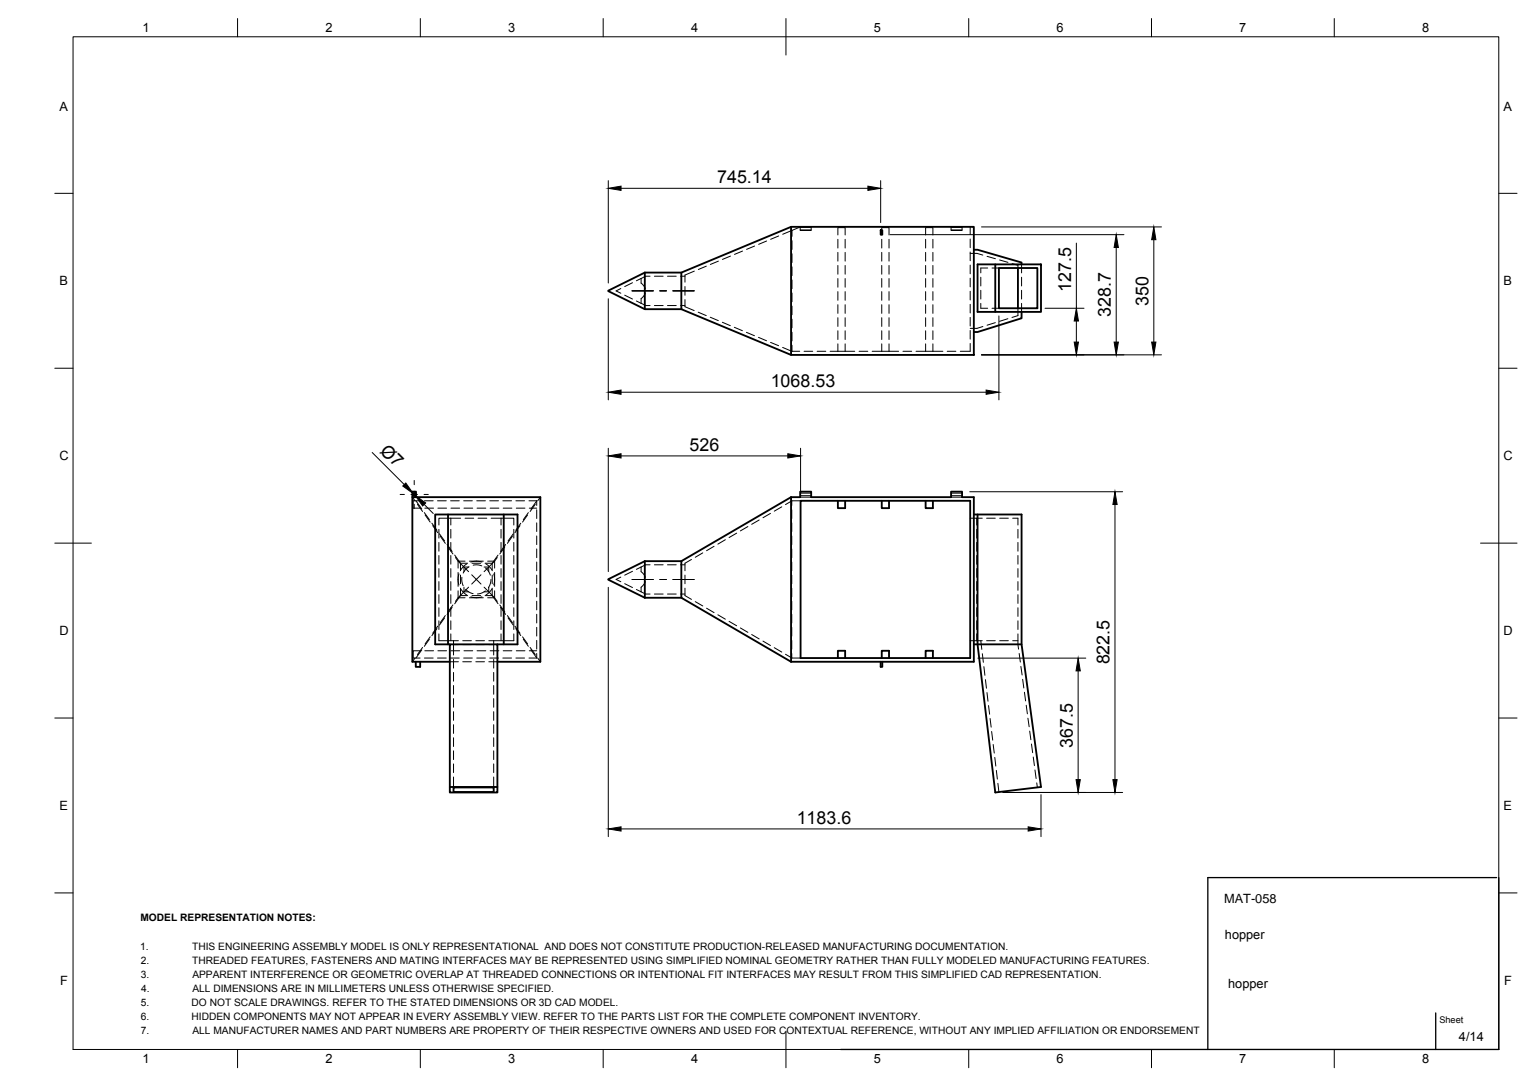
ISO-10303-21;
HEADER;
FILE_DESCRIPTION (('STEP AP214'),
    '1' );
FILE_NAME ('hopper.step',
    '2026-10-21T17:54:40',
    ( '' ),
    ( '' ),
    'SwSTEP 2.0',
    'SolidWorks 2026',
    '' );
FILE_SCHEMA (( 'AUTOMOTIVE_DESIGN' ));
ENDSEC;

DATA;
#6=ADVANCED_FACE ( 'NONE', ( #30321 ), #29814, .T. ) ;
#33=VECTOR ( 'NONE', #35078, 1000.000000000000000 ) ;
#69=AXIS2_PLACEMENT_3D ( 'NONE', #31209, #39422, #27614 ) ;
#97=LINE ( 'NONE', #40110, #967 ) ;
#99=ORIENTED_EDGE ( 'NONE', *, *, #35916, .T. ) ;
#106=CARTESIAN_POINT ( 'NONE',  ( -194.9999999999999432, 173.0000000000000000, 372.0000000000000000 ) ) ;
#168=ADVANCED_FACE ( 'NONE', ( #34691 ), #50265, .F. ) ;
#187=CARTESIAN_POINT ( 'NONE',  ( 214.9999999999999432, 164.9999999999999716, 132.0000000000000000 ) ) ;
#200=DIRECTION ( 'NONE',  ( -0.000000000000000000, -0.000000000000000000, 1.000000000000000000 ) ) ;
#209=VECTOR ( 'NONE', #36714, 1000.000000000000000 ) ;
#234=DIRECTION ( 'NONE',  ( -0.8962124318248270161, 0.000000000000000000, 0.4436251537532894806 ) ) ;
#244=PLANE ( 'NONE',  #29355 ) ;
#300=EDGE_CURVE ( 'NONE', #33060, #42445, #25916, .T. ) ;
#327=DIRECTION ( 'NONE',  ( 1.000000000000000000, 0.000000000000000000, -0.000000000000000000 ) ) ;
#337=CARTESIAN_POINT ( 'NONE',  ( 0.000000000000000000, 0.000000000000000000, 910.0000000000000000 ) ) ;
#341=PLANE ( 'NONE',  #14465 ) ;
#350=DIRECTION ( 'NONE',  ( -1.000000000000000000, -0.000000000000000000, -0.000000000000000000 ) ) ;
#356=DIRECTION ( 'NONE',  ( 0.000000000000000000, -1.000000000000000000, 0.000000000000000000 ) ) ;
#365=ORIENTED_EDGE ( 'NONE', *, *, #8301, .F. ) ;
#366=DIRECTION ( 'NONE',  ( 1.000000000000000000, 0.000000000000000000, 0.000000000000000000 ) ) ;
#369=CARTESIAN_POINT ( 'NONE',  ( -225.0000000000000568, -165.6999999999999602, 254.8599999999999852 ) ) ;
#377=DIRECTION ( 'NONE',  ( 0.000000000000000000, -0.000000000000000000, -1.000000000000000000 ) ) ;
#378=CARTESIAN_POINT ( 'NONE',  ( 0.5000000000000000000, -0.5000000000000000000, 1000.000000000000000 ) ) ;
#386=CARTESIAN_POINT ( 'NONE',  ( 0.000000000000000000, 0.000000000000000000, 910.0000000000000000 ) ) ;
#398=ORIENTED_EDGE ( 'NONE', *, *, #44450, .F. ) ;
#403=EDGE_LOOP ( 'NONE', ( #46548, #45741, #3676, #28607 ) ) ;
#410=PLANE ( 'NONE',  #69 ) ;
#412=ORIENTED_EDGE ( 'NONE', *, *, #15278, .F. ) ;
#422=DIRECTION ( 'NONE',  ( 0.000000000000000000, -1.000000000000000000, 1.822804496942679766E-16 ) ) ;
#453=EDGE_CURVE ( 'NONE', #46359, #24983, #8124, .T. ) ;
#480=PLANE ( 'NONE',  #30774 ) ;
#486=EDGE_CURVE ( 'NONE', #24711, #40831, #43254, .T. ) ;
#509=ADVANCED_FACE ( 'NONE', ( #12210 ), #8377, .F. ) ;
#518=CARTESIAN_POINT ( 'NONE',  ( -239.0000000000000853, -165.6999999999999602, 254.8599999999999852 ) ) ;
#522=LINE ( 'NONE', #27456, #25721 ) ;
#528=CARTESIAN_POINT ( 'NONE',  ( -194.9999999999999432, 0.000000000000000000, 0.000000000000000000 ) ) ;
#539=EDGE_CURVE ( 'NONE', #9223, #45368, #5772, .T. ) ;
#582=PLANE ( 'NONE',  #3188 ) ;
#594=DIRECTION ( 'NONE',  ( 0.000000000000000000, 1.000000000000000000, -0.000000000000000000 ) ) ;
#597=ORIENTED_EDGE ( 'NONE', *, *, #24654, .T. ) ;
#612=DIRECTION ( 'NONE',  ( 0.5038710255240859137, 0.000000000000000000, -0.8637789008984335659 ) ) ;
#622=DIRECTION ( 'NONE',  ( 0.000000000000000000, -1.000000000000000000, 0.000000000000000000 ) ) ;
#624=CARTESIAN_POINT ( 'NONE',  ( 432.7825420346616170, 74.83106485270648989, -130.5992382549688955 ) ) ;
#629=ADVANCED_FACE ( 'NONE', ( #5269 ), #9371, .F. ) ;
#639=VERTEX_POINT ( 'NONE', #48070 ) ;
#670=DIRECTION ( 'NONE',  ( -1.000000000000000000, 0.000000000000000000, 0.000000000000000000 ) ) ;
#671=LINE ( 'NONE', #11708, #25318 ) ;
#679=AXIS2_PLACEMENT_3D ( 'NONE', #33054, #24590, #40002 ) ;
#682=DIRECTION ( 'NONE',  ( 1.000000000000000000, 0.000000000000000000, 0.000000000000000000 ) ) ;
#684=ORIENTED_EDGE ( 'NONE', *, *, #22229, .T. ) ;
#707=CARTESIAN_POINT ( 'NONE',  ( 194.9999999999999432, 0.000000000000000000, 0.000000000000000000 ) ) ;
#708=DIRECTION ( 'NONE',  ( -1.000000000000000000, -0.000000000000000000, -0.000000000000000000 ) ) ;
#718=EDGE_CURVE ( 'NONE', #17041, #22983, #49580, .T. ) ;
#721=ORIENTED_EDGE ( 'NONE', *, *, #6928, .T. ) ;
#739=ADVANCED_FACE ( 'NONE', ( #38101 ), #2185, .F. ) ;
#759=CARTESIAN_POINT ( 'NONE',  ( 224.9999999999999716, -175.0000000000000000, 32.29650858650035161 ) ) ;
#777=EDGE_LOOP ( 'NONE', ( #3669, #1337, #39144 ) ) ;
#832=DIRECTION ( 'NONE',  ( -1.000000000000000000, 0.000000000000000000, -0.000000000000000000 ) ) ;
#835=VERTEX_POINT ( 'NONE', #19344 ) ;
#863=CARTESIAN_POINT ( 'NONE',  ( -582.5000000000000000, -62.49999999999998579, -58.60000000000003695 ) ) ;
#893=ADVANCED_FACE ( 'NONE', ( #43200 ), #31679, .T. ) ;
#916=VECTOR ( 'NONE', #24302, 1000.000000000000000 ) ;
#957=ORIENTED_EDGE ( 'NONE', *, *, #47722, .F. ) ;
#967=VECTOR ( 'NONE', #8554, 1000.000000000000000 ) ;
#968=AXIS2_PLACEMENT_3D ( 'NONE', #46813, #24023, #39678 ) ;
#998=ORIENTED_EDGE ( 'NONE', *, *, #4229, .F. ) ;
#1029=CARTESIAN_POINT ( 'NONE',  ( -177.4999999999999716, -112.5000000000000000, 0.000000000000000000 ) ) ;
#1031=LINE ( 'NONE', #47673, #2150 ) ;
#1101=EDGE_CURVE ( 'NONE', #1605, #16604, #6463, .T. ) ;
#1105=LINE ( 'NONE', #32921, #6079 ) ;
#1108=VERTEX_POINT ( 'NONE', #30327 ) ;
#1153=LINE ( 'NONE', #40404, #2135 ) ;
#1158=ADVANCED_FACE ( 'NONE', ( #25983 ), #18252, .T. ) ;
#1180=VERTEX_POINT ( 'NONE', #43137 ) ;
#1216=CARTESIAN_POINT ( 'NONE',  ( -194.9999999999999432, 173.0000000000000000, 372.0000000000000000 ) ) ;
#1223=EDGE_LOOP ( 'NONE', ( #7970, #34321, #34358, #11048, #18357 ) ) ;
#1239=DIRECTION ( 'NONE',  ( 0.000000000000000000, 1.000000000000000000, -1.604368532695312981E-16 ) ) ;
#1251=CARTESIAN_POINT ( 'NONE',  ( -194.9999999999999432, 173.0000000000000000, 352.0000000000000000 ) ) ;
#1277=VERTEX_POINT ( 'NONE', #31354 ) ;
#1294=CARTESIAN_POINT ( 'NONE',  ( -194.9999999999999432, -173.0000000000000000, 112.0000000000000284 ) ) ;
#1297=ORIENTED_EDGE ( 'NONE', *, *, #29279, .F. ) ;
#1320=VECTOR ( 'NONE', #10755, 1000.000000000000000 ) ;
#1322=FACE_OUTER_BOUND ( 'NONE', #22327, .T. ) ;
#1331=FACE_OUTER_BOUND ( 'NONE', #22843, .T. ) ;
#1337=ORIENTED_EDGE ( 'NONE', *, *, #38708, .T. ) ;
#1346=ORIENTED_EDGE ( 'NONE', *, *, #8118, .F. ) ;
#1366=ORIENTED_EDGE ( 'NONE', *, *, #27702, .T. ) ;
#1387=EDGE_CURVE ( 'NONE', #48005, #43486, #12216, .T. ) ;
#1404=ORIENTED_EDGE ( 'NONE', *, *, #36761, .F. ) ;
#1413=ORIENTED_EDGE ( 'NONE', *, *, #36701, .F. ) ;
#1417=APPLICATION_CONTEXT ( 'automotive_design' ) ;
#1422=EDGE_CURVE ( 'NONE', #29654, #38683, #36217, .T. ) ;
#1432=CARTESIAN_POINT ( 'NONE',  ( -239.0000000000000853, -153.6999999999999602, 250.3600000000000136 ) ) ;
#1451=EDGE_CURVE ( 'NONE', #40407, #50112, #29507, .T. ) ;
#1465=CARTESIAN_POINT ( 'NONE',  ( 0.000000000000000000, 0.000000000000000000, 900.0000000000000000 ) ) ;
#1505=ORIENTED_EDGE ( 'NONE', *, *, #34788, .T. ) ;
#1514=LINE ( 'NONE', #36425, #23413 ) ;
#1551=VERTEX_POINT ( 'NONE', #25409 ) ;
#1559=FACE_BOUND ( 'NONE', #31740, .T. ) ;
#1560=VECTOR ( 'NONE', #24107, 1000.000000000000000 ) ;
#1573=AXIS2_PLACEMENT_3D ( 'NONE', #18165, #48670, #2769 ) ;
#1579=ADVANCED_FACE ( 'NONE', ( #42810 ), #39243, .T. ) ;
#1598=CARTESIAN_POINT ( 'NONE',  ( -194.9999999999999432, 173.0000000000000000, 252.0000000000000000 ) ) ;
#1602=VECTOR ( 'NONE', #41002, 1000.000000000000000 ) ;
#1605=VERTEX_POINT ( 'NONE', #42557 ) ;
#1608=CARTESIAN_POINT ( 'NONE',  ( 214.9999999999999432, -173.0000000000000000, 352.0000000000001137 ) ) ;
#1619=DIRECTION ( 'NONE',  ( 0.000000000000000000, -0.3846153846153845812, -0.9230769230769231282 ) ) ;
#1638=PLANE ( 'NONE',  #22895 ) ;
#1664=EDGE_CURVE ( 'NONE', #10051, #46359, #30516, .T. ) ;
#1670=ORIENTED_EDGE ( 'NONE', *, *, #18646, .F. ) ;
#1671=ORIENTED_EDGE ( 'NONE', *, *, #6376, .T. ) ;
#1675=ORIENTED_EDGE ( 'NONE', *, *, #11798, .F. ) ;
#1677=LINE ( 'NONE', #29126, #7788 ) ;
#1700=EDGE_CURVE ( 'NONE', #4161, #27522, #26915, .T. ) ;
#1708=ORIENTED_EDGE ( 'NONE', *, *, #46797, .T. ) ;
#1717=VERTEX_POINT ( 'NONE', #3556 ) ;
#1747=EDGE_CURVE ( 'NONE', #14468, #4061, #20996, .T. ) ;
#1755=CARTESIAN_POINT ( 'NONE',  ( -40.00000000000000000, 7.564790863224932771, 897.6604670114604687 ) ) ;
#1769=ORIENTED_EDGE ( 'NONE', *, *, #14706, .T. ) ;
#1787=DIRECTION ( 'NONE',  ( 0.000000000000000000, 0.000000000000000000, 1.000000000000000000 ) ) ;
#1826=PLANE ( 'NONE',  #26243 ) ;
#1830=EDGE_LOOP ( 'NONE', ( #15260, #39633, #17503, #99 ) ) ;
#1840=EDGE_LOOP ( 'NONE', ( #2850, #9840, #48262, #41892 ) ) ;
#1848=CARTESIAN_POINT ( 'NONE',  ( 0.000000000000000000, 397.9839762253770346, 197.0020682315616796 ) ) ;
#1874=CARTESIAN_POINT ( 'NONE',  ( 224.9999999999999432, -175.0000000000000000, 500.0000000000000000 ) ) ;
#1891=LINE ( 'NONE', #18273, #4237 ) ;
#1934=VECTOR ( 'NONE', #20913, 1000.000000000000000 ) ;
#1949=VECTOR ( 'NONE', #31036, 1000.000000000000000 ) ;
#1971=CARTESIAN_POINT ( 'NONE',  ( 40.00000000000000000, 4.898587196589413026E-15, 897.6604670114603550 ) ) ;
#1990=PLANE ( 'NONE',  #14461 ) ;
#1995=CARTESIAN_POINT ( 'NONE',  ( 0.000000000000000000, -62.49999999999998579, 0.000000000000000000 ) ) ;
#2021=VERTEX_POINT ( 'NONE', #7112 ) ;
#2031=ORIENTED_EDGE ( 'NONE', *, *, #39450, .F. ) ;
#2065=ORIENTED_EDGE ( 'NONE', *, *, #1387, .F. ) ;
#2127=DIRECTION ( 'NONE',  ( 1.000000000000000000, -0.000000000000000000, -0.000000000000000000 ) ) ;
#2128=CARTESIAN_POINT ( 'NONE',  ( 224.9999999999999716, -164.9999999999999716, 444.9999999999998295 ) ) ;
#2133=PLANE ( 'NONE',  #45719 ) ;
#2135=VECTOR ( 'NONE', #16795, 1000.000000000000000 ) ;
#2142=ORIENTED_EDGE ( 'NONE', *, *, #40307, .F. ) ;
#2150=VECTOR ( 'NONE', #4374, 1000.000000000000000 ) ;
#2157=ORIENTED_EDGE ( 'NONE', *, *, #8118, .T. ) ;
#2159=CARTESIAN_POINT ( 'NONE',  ( -225.0000000000000568, 175.0000000000000000, 500.0000000000000000 ) ) ;
#2178=ORIENTED_EDGE ( 'NONE', *, *, #39801, .T. ) ;
#2185=PLANE ( 'NONE',  #27691 ) ;
#2192=CARTESIAN_POINT ( 'NONE',  ( 240.0000000000000000, -175.0000000000000000, 62.29650858650038003 ) ) ;
#2283=ORIENTED_EDGE ( 'NONE', *, *, #31995, .T. ) ;
#2295=ORIENTED_EDGE ( 'NONE', *, *, #4223, .T. ) ;
#2299=ORIENTED_EDGE ( 'NONE', *, *, #34194, .T. ) ;
#2311=( LENGTH_UNIT ( ) NAMED_UNIT ( * ) SI_UNIT ( .MILLI., .METRE. ) );
#2312=ORIENTED_EDGE ( 'NONE', *, *, #46993, .T. ) ;
#2325=ADVANCED_FACE ( 'NONE', ( #28785, #24942 ), #13863, .T. ) ;
#2334=ORIENTED_EDGE ( 'NONE', *, *, #7131, .T. ) ;
#2357=ORIENTED_EDGE ( 'NONE', *, *, #32200, .F. ) ;
#2380=EDGE_CURVE ( 'NONE', #47565, #36849, #41841, .T. ) ;
#2399=LINE ( 'NONE', #2159, #50424 ) ;
#2448=DIRECTION ( 'NONE',  ( -0.000000000000000000, 0.000000000000000000, 1.000000000000000000 ) ) ;
#2463=ORIENTED_EDGE ( 'NONE', *, *, #45939, .T. ) ;
#2475=EDGE_CURVE ( 'NONE', #11215, #9008, #2578, .T. ) ;
#2482=ORIENTED_EDGE ( 'NONE', *, *, #13416, .F. ) ;
#2486=EDGE_CURVE ( 'NONE', #29488, #7843, #23607, .T. ) ;
#2521=VERTEX_POINT ( 'NONE', #24134 ) ;
#2532=ORIENTED_EDGE ( 'NONE', *, *, #20272, .T. ) ;
#2537=ORIENTED_EDGE ( 'NONE', *, *, #31216, .T. ) ;
#2566=VERTEX_POINT ( 'NONE', #39026 ) ;
#2578=LINE ( 'NONE', #35436, #32315 ) ;
#2585=ORIENTED_EDGE ( 'NONE', *, *, #25789, .T. ) ;
#2595=AXIS2_PLACEMENT_3D ( 'NONE', #29831, #45444, #49528 ) ;
#2628=ADVANCED_FACE ( 'NONE', ( #7973 ), #4854, .T. ) ;
#2630=AXIS2_PLACEMENT_3D ( 'NONE', #12172, #28324, #12413 ) ;
#2631=EDGE_CURVE ( 'NONE', #31059, #39414, #19493, .T. ) ;
#2634=CARTESIAN_POINT ( 'NONE',  ( -177.4999999999999716, -112.5000000000000000, -9.999999999999973355 ) ) ;
#2640=EDGE_CURVE ( 'NONE', #12164, #16324, #41029, .T. ) ;
#2661=VECTOR ( 'NONE', #35085, 1000.000000000000000 ) ;
#2667=DIRECTION ( 'NONE',  ( 0.000000000000000000, 0.000000000000000000, -1.000000000000000000 ) ) ;
#2681=CARTESIAN_POINT ( 'NONE',  ( 33.89193117067290473, 0.000000000000000000, 910.0000000000000000 ) ) ;
#2710=DIRECTION ( 'NONE',  ( -0.000000000000000000, 0.000000000000000000, -1.000000000000000000 ) ) ;
#2713=VERTEX_POINT ( 'NONE', #32588 ) ;
#2730=CYLINDRICAL_SURFACE ( 'NONE', #5117, 50.00000000000000000 ) ;
#2739=DIRECTION ( 'NONE',  ( -0.000000000000000000, 1.000000000000000000, -1.604368532695312981E-16 ) ) ;
#2740=FACE_OUTER_BOUND ( 'NONE', #48298, .T. ) ;
#2769=DIRECTION ( 'NONE',  ( 0.4436251537532894806, 0.000000000000000000, -0.8962124318248270161 ) ) ;
#2775=LINE ( 'NONE', #31012, #29883 ) ;
#2798=EDGE_LOOP ( 'NONE', ( #14811, #28770, #6712, #21908, #31731, #40300, #17842, #23739, #30597, #13220, #37844, #41783 ) ) ;
#2817=EDGE_LOOP ( 'NONE', ( #412, #31040, #39958, #40471 ) ) ;
#2824=CARTESIAN_POINT ( 'NONE',  ( 40.00000000000000000, 4.898587196589413026E-15, 900.0000000000000000 ) ) ;
#2825=DIRECTION ( 'NONE',  ( 0.000000000000000000, -0.4436251537532894806, -0.8962124318248270161 ) ) ;
#2828=CARTESIAN_POINT ( 'NONE',  ( 177.5000000000000284, -112.5000000000000000, 0.000000000000000000 ) ) ;
#2830=ORIENTED_EDGE ( 'NONE', *, *, #4563, .T. ) ;
#2835=CARTESIAN_POINT ( 'NONE',  ( 240.0000000000000000, -164.9999999999999716, 32.29650858650035161 ) ) ;
#2850=ORIENTED_EDGE ( 'NONE', *, *, #28204, .F. ) ;
#2866=AXIS2_PLACEMENT_3D ( 'NONE', #16122, #31532, #31277 ) ;
#2887=DIRECTION ( 'NONE',  ( 1.000000000000000000, 0.000000000000000000, 0.000000000000000000 ) ) ;
#2901=VECTOR ( 'NONE', #12023, 1000.000000000000000 ) ;
#2925=LINE ( 'NONE', #2681, #43678 ) ;
#2931=CARTESIAN_POINT ( 'NONE',  ( -225.0000000000000568, 164.9999999999999716, 372.0000000000000000 ) ) ;
#2992=DIRECTION ( 'NONE',  ( 0.000000000000000000, -0.000000000000000000, 1.000000000000000000 ) ) ;
#3002=CARTESIAN_POINT ( 'NONE',  ( 224.9999999999999716, -175.0000000000000000, 62.29650858650038003 ) ) ;
#3020=EDGE_CURVE ( 'NONE', #4421, #16851, #21653, .T. ) ;
#3034=EDGE_LOOP ( 'NONE', ( #18109, #6648, #12703, #38229 ) ) ;
#3047=DIRECTION ( 'NONE',  ( 0.000000000000000000, -1.000000000000000000, 0.000000000000000000 ) ) ;
#3073=ORIENTED_EDGE ( 'NONE', *, *, #30278, .T. ) ;
#3081=DIRECTION ( 'NONE',  ( 0.000000000000000000, 0.000000000000000000, -1.000000000000000000 ) ) ;
#3123=DIRECTION ( 'NONE',  ( 0.5038710255240859137, 0.000000000000000000, -0.8637789008984335659 ) ) ;
#3164=DIRECTION ( 'NONE',  ( 0.000000000000000000, 1.000000000000000000, 0.000000000000000000 ) ) ;
#3188=AXIS2_PLACEMENT_3D ( 'NONE', #32896, #16223, #832 ) ;
#3191=LINE ( 'NONE', #10905, #28331 ) ;
#3201=CARTESIAN_POINT ( 'NONE',  ( 50.00000000000000000, -50.00000000000000000, 800.0000000000000000 ) ) ;
#3211=VERTEX_POINT ( 'NONE', #39099 ) ;
#3218=CIRCLE ( 'NONE', #48246, 50.00000000000000000 ) ;
#3230=ADVANCED_FACE ( 'NONE', ( #19562, #27282 ), #42658, .F. ) ;
#3255=LINE ( 'NONE', #34087, #25681 ) ;
#3261=EDGE_CURVE ( 'NONE', #43354, #4645, #14712, .T. ) ;
#3270=CARTESIAN_POINT ( 'NONE',  ( 194.9999999999999432, -173.0000000000000000, 112.0000000000000284 ) ) ;
#3281=DIRECTION ( 'NONE',  ( -0.000000000000000000, 0.000000000000000000, 1.000000000000000000 ) ) ;
#3326=EDGE_CURVE ( 'NONE', #4061, #30057, #32145, .T. ) ;
#3345=ORIENTED_EDGE ( 'NONE', *, *, #30501, .F. ) ;
#3378=CARTESIAN_POINT ( 'NONE',  ( 194.9999999999999432, -172.9999999999999716, 232.0000000000000284 ) ) ;
#3398=CARTESIAN_POINT ( 'NONE',  ( 194.9999999999999432, -172.9999999999999716, 232.0000000000000284 ) ) ;
#3418=ORIENTED_EDGE ( 'NONE', *, *, #45707, .T. ) ;
#3419=CARTESIAN_POINT ( 'NONE',  ( -225.0000000000000568, -165.6999999999999602, 250.3600000000000136 ) ) ;
#3424=ORIENTED_EDGE ( 'NONE', *, *, #3949, .T. ) ;
#3433=FACE_OUTER_BOUND ( 'NONE', #13573, .T. ) ;
#3444=CARTESIAN_POINT ( 'NONE',  ( 236.0000000000000000, -169.9999999999999716, 32.29650858650035161 ) ) ;
#3448=FACE_OUTER_BOUND ( 'NONE', #48944, .T. ) ;
#3475=DIRECTION ( 'NONE',  ( 0.000000000000000000, 1.000000000000000000, -1.604368532695312981E-16 ) ) ;
#3500=DIRECTION ( 'NONE',  ( 0.000000000000000000, -1.000000000000000000, 0.000000000000000000 ) ) ;
#3507=LINE ( 'NONE', #30472, #28266 ) ;
#3528=ORIENTED_EDGE ( 'NONE', *, *, #11798, .T. ) ;
#3531=ORIENTED_EDGE ( 'NONE', *, *, #18390, .T. ) ;
#3556=CARTESIAN_POINT ( 'NONE',  ( 194.9999999999999432, 164.9999999999999716, 231.9999999999999716 ) ) ;
#3559=ADVANCED_FACE ( 'NONE', ( #40598 ), #5433, .T. ) ;
#3562=DIRECTION ( 'NONE',  ( 0.000000000000000000, -0.000000000000000000, -1.000000000000000000 ) ) ;
#3565=DIRECTION ( 'NONE',  ( -0.000000000000000000, -0.000000000000000000, 1.000000000000000000 ) ) ;
#3581=EDGE_CURVE ( 'NONE', #12455, #37995, #22343, .T. ) ;
#3588=FACE_OUTER_BOUND ( 'NONE', #35618, .T. ) ;
#3592=CARTESIAN_POINT ( 'NONE',  ( 194.9999999999999432, -173.0000000000000000, 352.0000000000000568 ) ) ;
#3623=VERTEX_POINT ( 'NONE', #2835 ) ;
#3652=ADVANCED_FACE ( 'NONE', ( #30064 ), #10795, .T. ) ;
#3662=FACE_OUTER_BOUND ( 'NONE', #50102, .T. ) ;
#3669=ORIENTED_EDGE ( 'NONE', *, *, #30323, .F. ) ;
#3676=ORIENTED_EDGE ( 'NONE', *, *, #44948, .F. ) ;
#3691=EDGE_CURVE ( 'NONE', #24521, #30113, #20524, .T. ) ;
#3695=ORIENTED_EDGE ( 'NONE', *, *, #39267, .F. ) ;
#3696=ORIENTED_EDGE ( 'NONE', *, *, #21537, .F. ) ;
#3700=EDGE_CURVE ( 'NONE', #40759, #18948, #23685, .T. ) ;
#3737=CARTESIAN_POINT ( 'NONE',  ( -40.00000000000000000, 0.000000000000000000, 897.6604670114603550 ) ) ;
#3740=CARTESIAN_POINT ( 'NONE',  ( 40.00000000000000000, 4.898587196589413026E-15, 897.6604670114603550 ) ) ;
#3749=CARTESIAN_POINT ( 'NONE',  ( -7.884183412771418986, 42.26678417219199702, 893.0811050474360400 ) ) ;
#3753=CARTESIAN_POINT ( 'NONE',  ( -194.9999999999999432, -173.0000000000000000, 112.0000000000000284 ) ) ;
#3762=DIRECTION ( 'NONE',  ( -0.000000000000000000, 0.000000000000000000, 1.000000000000000000 ) ) ;
#3778=EDGE_LOOP ( 'NONE', ( #35698, #6071, #6455, #44785 ) ) ;
#3788=VECTOR ( 'NONE', #45975, 1000.000000000000114 ) ;
#3828=EDGE_CURVE ( 'NONE', #36764, #21950, #24141, .T. ) ;
#3860=ORIENTED_EDGE ( 'NONE', *, *, #31285, .F. ) ;
#3870=CYLINDRICAL_SURFACE ( 'NONE', #45910, 3.500000000000003109 ) ;
#3898=PLANE ( 'NONE',  #36039 ) ;
#3900=LINE ( 'NONE', #15702, #48312 ) ;
#3907=PLANE ( 'NONE',  #42666 ) ;
#3920=ORIENTED_EDGE ( 'NONE', *, *, #13177, .F. ) ;
#3947=LINE ( 'NONE', #32669, #24210 ) ;
#3949=EDGE_CURVE ( 'NONE', #7843, #1108, #14331, .T. ) ;
#3953=DIRECTION ( 'NONE',  ( 1.000000000000000000, 0.000000000000000000, 0.000000000000000000 ) ) ;
#3957=CARTESIAN_POINT ( 'NONE',  ( -214.9999999999999432, 173.0000000000000000, 352.0000000000000000 ) ) ;
#3960=EDGE_CURVE ( 'NONE', #43789, #4257, #22791, .T. ) ;
#3968=CARTESIAN_POINT ( 'NONE',  ( 194.9999999999999432, -173.0000000000000000, 352.0000000000000568 ) ) ;
#3989=EDGE_CURVE ( 'NONE', #2713, #24145, #14585, .T. ) ;
#4015=VECTOR ( 'NONE', #3281, 1000.000000000000000 ) ;
#4018=DIRECTION ( 'NONE',  ( 1.000000000000000000, 0.000000000000000000, 0.000000000000000000 ) ) ;
#4041=CIRCLE ( 'NONE', #7336, 3.500000000000003109 ) ;
#4045=ORIENTED_EDGE ( 'NONE', *, *, #1422, .F. ) ;
#4061=VERTEX_POINT ( 'NONE', #26650 ) ;
#4066=DIRECTION ( 'NONE',  ( 0.000000000000000000, 1.000000000000000000, 0.000000000000000000 ) ) ;
#4118=VECTOR ( 'NONE', #13988, 1000.000000000000000 ) ;
#4123=VECTOR ( 'NONE', #17070, 1000.000000000000227 ) ;
#4161=VERTEX_POINT ( 'NONE', #19707 ) ;
#4169=CARTESIAN_POINT ( 'NONE',  ( -215.0000000000000568, 164.9999999999999716, 500.0000000000000000 ) ) ;
#4174=CARTESIAN_POINT ( 'NONE',  ( 0.000000000000000000, 317.3964497041420145, 132.2485207100591253 ) ) ;
#4203=ORIENTED_EDGE ( 'NONE', *, *, #5443, .T. ) ;
#4206=ORIENTED_EDGE ( 'NONE', *, *, #20417, .T. ) ;
#4217=DIRECTION ( 'NONE',  ( 0.000000000000000000, -1.000000000000000000, 0.000000000000000000 ) ) ;
#4223=EDGE_CURVE ( 'NONE', #43883, #12455, #35884, .T. ) ;
#4228=DIRECTION ( 'NONE',  ( -0.000000000000000000, -0.000000000000000000, 1.000000000000000000 ) ) ;
#4229=EDGE_CURVE ( 'NONE', #16113, #9008, #3218, .T. ) ;
#4237=VECTOR ( 'NONE', #49541, 1000.000000000000000 ) ;
#4244=ORIENTED_EDGE ( 'NONE', *, *, #18390, .F. ) ;
#4246=DIRECTION ( 'NONE',  ( 1.000000000000000000, -0.000000000000000000, -0.000000000000000000 ) ) ;
#4247=DIRECTION ( 'NONE',  ( 1.000000000000000000, 0.000000000000000000, 0.000000000000000000 ) ) ;
#4257=VERTEX_POINT ( 'NONE', #38968 ) ;
#4276=DIRECTION ( 'NONE',  ( 0.4740998230350172427, -0.3386427307392981811, -0.8127425537743158124 ) ) ;
#4306=DIRECTION ( 'NONE',  ( 0.000000000000000000, 1.000000000000000000, 0.000000000000000000 ) ) ;
#4329=DIRECTION ( 'NONE',  ( 0.4436251537532894806, 0.000000000000000000, 0.8962124318248270161 ) ) ;
#4374=DIRECTION ( 'NONE',  ( -0.000000000000000000, -0.000000000000000000, 1.000000000000000000 ) ) ;
#4405=DIRECTION ( 'NONE',  ( -1.000000000000000000, 0.000000000000000000, 0.000000000000000000 ) ) ;
#4412=ADVANCED_FACE ( 'NONE', ( #25833 ), #26587, .F. ) ;
#4420=CARTESIAN_POINT ( 'NONE',  ( -194.9999999999999432, 173.0000000000000000, 352.0000000000000000 ) ) ;
#4421=VERTEX_POINT ( 'NONE', #18617 ) ;
#4453=FACE_OUTER_BOUND ( 'NONE', #30124, .T. ) ;
#4465=CARTESIAN_POINT ( 'NONE',  ( 224.9999999999999432, -175.0000000000000000, 0.000000000000000000 ) ) ;
#4466=FACE_OUTER_BOUND ( 'NONE', #46897, .T. ) ;
#4478=ADVANCED_FACE ( 'NONE', ( #11959 ), #410, .T. ) ;
#4495=VERTEX_POINT ( 'NONE', #7864 ) ;
#4516=DIRECTION ( 'NONE',  ( -1.000000000000000000, -0.000000000000000000, -0.000000000000000000 ) ) ;
#4517=DIRECTION ( 'NONE',  ( -0.000000000000000000, -0.000000000000000000, -1.000000000000000000 ) ) ;
#4526=AXIS2_PLACEMENT_3D ( 'NONE', #4542, #24311, #17847 ) ;
#4542=CARTESIAN_POINT ( 'NONE',  ( -567.5000000000000000, 57.49999999999996447, -183.5999999999997954 ) ) ;
#4548=CARTESIAN_POINT ( 'NONE',  ( 214.9999999999999432, 164.9999999999999716, 10.00000000000000000 ) ) ;
#4559=CARTESIAN_POINT ( 'NONE',  ( -50.00000000000000000, 50.00000000000000000, 800.0000000000000000 ) ) ;
#4563=EDGE_CURVE ( 'NONE', #19653, #1180, #33919, .T. ) ;
#4581=CARTESIAN_POINT ( 'NONE',  ( 214.9999999999999432, -173.0000000000000000, 111.9999999999999858 ) ) ;
#4602=VERTEX_POINT ( 'NONE', #45421 ) ;
#4603=VECTOR ( 'NONE', #23093, 1000.000000000000114 ) ;
#4632=CARTESIAN_POINT ( 'NONE',  ( -239.0000000000000853, -153.6999999999999602, 254.8599999999999852 ) ) ;
#4645=VERTEX_POINT ( 'NONE', #5000 ) ;
#4671=CARTESIAN_POINT ( 'NONE',  ( -225.0000000000000568, -175.0000000000000000, 474.0000000000000000 ) ) ;
#4694=ORIENTED_EDGE ( 'NONE', *, *, #24357, .F. ) ;
#4723=LINE ( 'NONE', #28068, #49597 ) ;
#4729=ORIENTED_EDGE ( 'NONE', *, *, #33672, .F. ) ;
#4750=PLANE ( 'NONE',  #34099 ) ;
#4755=ADVANCED_FACE ( 'NONE', ( #42858 ), #3870, .F. ) ;
#4757=CARTESIAN_POINT ( 'NONE',  ( -239.0000000000000853, -165.6999999999999602, 250.3600000000000136 ) ) ;
#4767=DIRECTION ( 'NONE',  ( 0.000000000000000000, 0.2981428420003837121, 0.9545212652235329776 ) ) ;
#4796=EDGE_LOOP ( 'NONE', ( #46929, #32323, #13463, #23269, #24151, #2295, #23463, #49917, #30279, #15234, #47814, #24622, #25644, #5470, #684, #2532, #10930 ) ) ;
#4806=CARTESIAN_POINT ( 'NONE',  ( 224.9999999999999716, -175.0000000000000000, 474.9999999999998863 ) ) ;
#4811=ADVANCED_FACE ( 'NONE', ( #11578 ), #42097, .T. ) ;
#4818=CARTESIAN_POINT ( 'NONE',  ( -194.9999999999999432, -173.0000000000000000, 132.0000000000000853 ) ) ;
#4839=LINE ( 'NONE', #13296, #28132 ) ;
#4840=VECTOR ( 'NONE', #10206, 1000.000000000000000 ) ;
#4854=PLANE ( 'NONE',  #31475 ) ;
#4869=AXIS2_PLACEMENT_3D ( 'NONE', #10277, #33888, #49481 ) ;
#4870=LINE ( 'NONE', #28242, #50272 ) ;
#4879=( BOUNDED_CURVE ( )  B_SPLINE_CURVE ( 3, ( #15037, #18616, #27613, #3740 ),
 .UNSPECIFIED., .F., .F. ) 
 B_SPLINE_CURVE_WITH_KNOTS ( ( 4, 4 ),
 ( 5.723266580096324496, 6.283185307179586232 ),
 .UNSPECIFIED. ) 
 CURVE ( )  GEOMETRIC_REPRESENTATION_ITEM ( )  RATIONAL_B_SPLINE_CURVE ( ( 1.000000000000000000, 0.9740444450880465510, 0.9740444450880465510, 1.000000000000000000 ) ) 
 REPRESENTATION_ITEM ( '' )  );
#4887=EDGE_CURVE ( 'NONE', #9722, #32176, #8748, .T. ) ;
#4888=CARTESIAN_POINT ( 'NONE',  ( -177.4999999999999716, 57.49999999999996447, -130.5992382549688671 ) ) ;
#4939=ORIENTED_EDGE ( 'NONE', *, *, #32846, .F. ) ;
#4966=DIRECTION ( 'NONE',  ( 0.000000000000000000, 0.000000000000000000, -1.000000000000000000 ) ) ;
#4969=DIRECTION ( 'NONE',  ( -0.000000000000000000, 0.000000000000000000, 1.000000000000000000 ) ) ;
#4986=VECTOR ( 'NONE', #39844, 1000.000000000000000 ) ;
#4992=CARTESIAN_POINT ( 'NONE',  ( 224.9999999999999716, -164.9999999999999716, 474.9999999999998863 ) ) ;
#4994=APPLICATION_CONTEXT ( 'automotive_design' ) ;
#5000=CARTESIAN_POINT ( 'NONE',  ( 214.5896300087916302, 164.9999999999999716, 498.0000000000001137 ) ) ;
#5008=EDGE_CURVE ( 'NONE', #29800, #22662, #9994, .T. ) ;
#5018=PLANE ( 'NONE',  #17902 ) ;
#5022=PLANE ( 'NONE',  #32724 ) ;
#5026=VERTEX_POINT ( 'NONE', #11003 ) ;
#5054=AXIS2_PLACEMENT_3D ( 'NONE', #46257, #4217, #377 ) ;
#5057=ORIENTED_EDGE ( 'NONE', *, *, #34937, .F. ) ;
#5058=ORIENTED_EDGE ( 'NONE', *, *, #11541, .T. ) ;
#5061=VERTEX_POINT ( 'NONE', #11515 ) ;
#5065=LINE ( 'NONE', #49323, #10838 ) ;
#5066=FACE_OUTER_BOUND ( 'NONE', #19576, .T. ) ;
#5085=VECTOR ( 'NONE', #35941, 1000.000000000000000 ) ;
#5109=EDGE_CURVE ( 'NONE', #44615, #44330, #30011, .T. ) ;
#5117=AXIS2_PLACEMENT_3D ( 'NONE', #11211, #26349, #18377 ) ;
#5152=EDGE_CURVE ( 'NONE', #39676, #9652, #15872, .T. ) ;
#5156=ORIENTED_EDGE ( 'NONE', *, *, #11085, .F. ) ;
#5192=LINE ( 'NONE', #16998, #17585 ) ;
#5196=ORIENTED_EDGE ( 'NONE', *, *, #14651, .F. ) ;
#5210=VERTEX_POINT ( 'NONE', #17630 ) ;
#5213=DIRECTION ( 'NONE',  ( -0.000000000000000000, -0.000000000000000000, 1.000000000000000000 ) ) ;
#5234=DIRECTION ( 'NONE',  ( 0.000000000000000000, 1.604368532695312981E-16, 1.000000000000000000 ) ) ;
#5254=EDGE_CURVE ( 'NONE', #27283, #42074, #29435, .T. ) ;
#5255=DIRECTION ( 'NONE',  ( -1.000000000000000000, 0.000000000000000000, 0.000000000000000000 ) ) ;
#5260=LINE ( 'NONE', #4757, #1934 ) ;
#5269=FACE_OUTER_BOUND ( 'NONE', #43195, .T. ) ;
#5290=CIRCLE ( 'NONE', #40536, 3.500000000000003109 ) ;
#5319=CARTESIAN_POINT ( 'NONE',  ( -214.9999999999999432, -172.9999999999999716, 232.0000000000000284 ) ) ;
#5320=DIRECTION ( 'NONE',  ( -1.000000000000000000, -0.000000000000000000, -0.000000000000000000 ) ) ;
#5321=ORIENTED_EDGE ( 'NONE', *, *, #26939, .T. ) ;
#5357=ADVANCED_FACE ( 'NONE', ( #36667 ), #2730, .T. ) ;
#5366=VECTOR ( 'NONE', #36991, 1000.000000000000000 ) ;
#5389=LINE ( 'NONE', #13830, #33860 ) ;
#5390=ORIENTED_EDGE ( 'NONE', *, *, #47503, .F. ) ;
#5394=DIRECTION ( 'NONE',  ( 0.000000000000000000, 0.000000000000000000, -1.000000000000000000 ) ) ;
#5414=CARTESIAN_POINT ( 'NONE',  ( -325.0507910275983932, 325.0507910275983932, 321.8002831173224649 ) ) ;
#5424=CARTESIAN_POINT ( 'NONE',  ( -167.4999999999999432, -102.5000000000000142, -8.575805527524005711 ) ) ;
#5429=VECTOR ( 'NONE', #4247, 1000.000000000000000 ) ;
#5433=PLANE ( 'NONE',  #14146 ) ;
#5443=EDGE_CURVE ( 'NONE', #31445, #37995, #45558, .T. ) ;
#5449=EDGE_CURVE ( 'NONE', #35427, #5026, #34826, .T. ) ;
#5467=FACE_OUTER_BOUND ( 'NONE', #2798, .T. ) ;
#5470=ORIENTED_EDGE ( 'NONE', *, *, #2631, .T. ) ;
#5477=EDGE_CURVE ( 'NONE', #24521, #41260, #28118, .T. ) ;
#5533=EDGE_CURVE ( 'NONE', #43883, #43789, #47322, .T. ) ;
#5545=EDGE_CURVE ( 'NONE', #14442, #45963, #40681, .T. ) ;
#5602=ORIENTED_EDGE ( 'NONE', *, *, #22353, .F. ) ;
#5614=EDGE_CURVE ( 'NONE', #2521, #44090, #20663, .T. ) ;
#5618=EDGE_LOOP ( 'NONE', ( #27292, #2178, #12293, #31627 ) ) ;
#5636=ADVANCED_FACE ( 'NONE', ( #38098 ), #6780, .F. ) ;
#5641=EDGE_LOOP ( 'NONE', ( #47808, #1671, #8547, #43786 ) ) ;
#5645=CARTESIAN_POINT ( 'NONE',  ( -239.0000000000000853, -153.6999999999999602, 250.3600000000000136 ) ) ;
#5673=DIRECTION ( 'NONE',  ( -0.000000000000000000, -0.000000000000000000, 1.000000000000000000 ) ) ;
#5677=ORIENTED_EDGE ( 'NONE', *, *, #49840, .F. ) ;
#5688=VECTOR ( 'NONE', #36681, 1000.000000000000000 ) ;
#5697=EDGE_LOOP ( 'NONE', ( #6929, #6365, #37231, #15190 ) ) ;
#5704=ORIENTED_EDGE ( 'NONE', *, *, #13082, .T. ) ;
#5714=PLANE ( 'NONE',  #2595 ) ;
#5717=VECTOR ( 'NONE', #37692, 1000.000000000000000 ) ;
#5746=CARTESIAN_POINT ( 'NONE',  ( -50.00000000000000000, -50.00000000000000000, 800.0000000000000000 ) ) ;
#5772=LINE ( 'NONE', #20665, #4123 ) ;
#5774=CARTESIAN_POINT ( 'NONE',  ( 167.4999999999999716, -102.8976013127941656, -7.208237214241163926 ) ) ;
#5778=EDGE_CURVE ( 'NONE', #13610, #17677, #30548, .T. ) ;
#5798=CARTESIAN_POINT ( 'NONE',  ( -568.8466156985925863, 47.50000000000000000, -173.6910835022032700 ) ) ;
#5805=ORIENTED_EDGE ( 'NONE', *, *, #47503, .T. ) ;
#5808=LINE ( 'NONE', #22463, #34488 ) ;
#5811=CARTESIAN_POINT ( 'NONE',  ( -239.0000000000000853, -165.6999999999999602, 250.3600000000000136 ) ) ;
#5842=PLANE ( 'NONE',  #26439 ) ;
#5843=VECTOR ( 'NONE', #30463, 1000.000000000000000 ) ;
#5852=ORIENTED_EDGE ( 'NONE', *, *, #3020, .T. ) ;
#5876=DIRECTION ( 'NONE',  ( 0.000000000000000000, -1.822804496942679766E-16, -1.000000000000000000 ) ) ;
#5902=CIRCLE ( 'NONE', #21462, 50.00000000000000000 ) ;
#5927=CIRCLE ( 'NONE', #12481, 40.00000000000000000 ) ;
#5942=DIRECTION ( 'NONE',  ( 0.000000000000000000, 0.000000000000000000, 1.000000000000000000 ) ) ;
#5946=LINE ( 'NONE', #13389, #42147 ) ;
#5950=MANIFOLD_SOLID_BREP ( 'Mirror1', #35140 ) ;
#5951=CARTESIAN_POINT ( 'NONE',  ( -397.9839762253770346, 0.000000000000000000, 197.0020682315616796 ) ) ;
#5967=DIRECTION ( 'NONE',  ( 1.000000000000000000, 0.000000000000000000, 0.000000000000000000 ) ) ;
#6025=CARTESIAN_POINT ( 'NONE',  ( 232.4999999999999716, -169.9999999999999716, 4.999999999999616307 ) ) ;
#6041=VECTOR ( 'NONE', #45873, 1000.000000000000000 ) ;
#6068=EDGE_LOOP ( 'NONE', ( #16968, #18794, #14384, #46517, #24022, #25623 ) ) ;
#6071=ORIENTED_EDGE ( 'NONE', *, *, #300, .T. ) ;
#6076=DIRECTION ( 'NONE',  ( 1.000000000000000000, -0.000000000000000000, 0.000000000000000000 ) ) ;
#6079=VECTOR ( 'NONE', #25455, 1000.000000000000000 ) ;
#6090=CARTESIAN_POINT ( 'NONE',  ( 44.25629667545849344, -43.33333333333335702, 790.0000000000000000 ) ) ;
#6096=VECTOR ( 'NONE', #16521, 1000.000000000000000 ) ;
#6098=VECTOR ( 'NONE', #13478, 1000.000000000000000 ) ;
#6115=ORIENTED_EDGE ( 'NONE', *, *, #7131, .F. ) ;
#6180=AXIS2_PLACEMENT_3D ( 'NONE', #12584, #5394, #32874 ) ;
#6186=EDGE_CURVE ( 'NONE', #33652, #36453, #18067, .T. ) ;
#6203=CARTESIAN_POINT ( 'NONE',  ( 0.000000000000000000, 0.000000000000000000, 900.0000000000000000 ) ) ;
#6216=ORIENTED_EDGE ( 'NONE', *, *, #14706, .F. ) ;
#6253=AXIS2_PLACEMENT_3D ( 'NONE', #13574, #44106, #24638 ) ;
#6254=DIRECTION ( 'NONE',  ( 0.000000000000000000, 0.000000000000000000, -1.000000000000000000 ) ) ;
#6267=ORIENTED_EDGE ( 'NONE', *, *, #34937, .T. ) ;
#6274=ORIENTED_EDGE ( 'NONE', *, *, #28678, .T. ) ;
#6295=CARTESIAN_POINT ( 'NONE',  ( -568.8466156985925863, -62.49999999999998579, -173.6910835022032700 ) ) ;
#6307=PLANE ( 'NONE',  #47557 ) ;
#6315=ORIENTED_EDGE ( 'NONE', *, *, #12252, .T. ) ;
#6320=ORIENTED_EDGE ( 'NONE', *, *, #28791, .F. ) ;
#6325=EDGE_CURVE ( 'NONE', #28214, #37651, #18397, .T. ) ;
#6337=LINE ( 'NONE', #49875, #38985 ) ;
#6352=DIRECTION ( 'NONE',  ( 0.000000000000000000, 0.000000000000000000, 1.000000000000000000 ) ) ;
#6362=VERTEX_POINT ( 'NONE', #34575 ) ;
#6364=ORIENTED_EDGE ( 'NONE', *, *, #1664, .T. ) ;
#6365=ORIENTED_EDGE ( 'NONE', *, *, #486, .F. ) ;
#6369=PLANE ( 'NONE',  #21284 ) ;
#6376=EDGE_CURVE ( 'NONE', #8986, #14100, #49662, .T. ) ;
#6409=ORIENTED_EDGE ( 'NONE', *, *, #44460, .F. ) ;
#6422=ORIENTED_EDGE ( 'NONE', *, *, #44926, .T. ) ;
#6428=EDGE_CURVE ( 'NONE', #7894, #36027, #35357, .T. ) ;
#6437=VERTEX_POINT ( 'NONE', #23783 ) ;
#6455=ORIENTED_EDGE ( 'NONE', *, *, #28927, .T. ) ;
#6463=LINE ( 'NONE', #18512, #39258 ) ;
#6465=CARTESIAN_POINT ( 'NONE',  ( 177.5000000000000284, 112.5000000000000000, -10.00000000000000000 ) ) ;
#6494=VECTOR ( 'NONE', #37963, 1000.000000000000000 ) ;
#6518=LINE ( 'NONE', #36668, #14947 ) ;
#6548=EDGE_CURVE ( 'NONE', #27522, #37293, #44018, .T. ) ;
#6622=CARTESIAN_POINT ( 'NONE',  ( -194.9999999999999432, 164.9999999999999716, 352.0000000000000000 ) ) ;
#6636=CARTESIAN_POINT ( 'NONE',  ( -177.4999999999999716, 74.83106485270648989, -130.5992382549688955 ) ) ;
#6642=DIRECTION ( 'NONE',  ( 0.000000000000000000, -0.2791762785758810650, 0.9602398687205827565 ) ) ;
#6648=ORIENTED_EDGE ( 'NONE', *, *, #4887, .F. ) ;
#6684=CARTESIAN_POINT ( 'NONE',  ( -176.3085477938156487, 47.50000000000000000, -19.92876838486919411 ) ) ;
#6712=ORIENTED_EDGE ( 'NONE', *, *, #29955, .T. ) ;
#6713=ADVANCED_FACE ( 'NONE', ( #41699 ), #14496, .F. ) ;
#6732=VECTOR ( 'NONE', #40922, 1000.000000000000000 ) ;
#6735=DIRECTION ( 'NONE',  ( 0.000000000000000000, -1.000000000000000000, 0.000000000000000000 ) ) ;
#6736=VECTOR ( 'NONE', #27929, 1000.000000000000000 ) ;
#6761=ADVANCED_FACE ( 'NONE', ( #6800, #22447 ), #6307, .T. ) ;
#6762=ORIENTED_EDGE ( 'NONE', *, *, #21537, .T. ) ;
#6765=EDGE_CURVE ( 'NONE', #24983, #41718, #10144, .T. ) ;
#6775=EDGE_LOOP ( 'NONE', ( #8519, #20508, #12338, #1769, #5058 ) ) ;
#6780=PLANE ( 'NONE',  #14978 ) ;
#6789=DIRECTION ( 'NONE',  ( 1.000000000000000000, 0.000000000000000000, 0.000000000000000000 ) ) ;
#6800=FACE_BOUND ( 'NONE', #36001, .T. ) ;
#6828=ADVANCED_FACE ( 'NONE', ( #8333 ), #11668, .F. ) ;
#6866=VECTOR ( 'NONE', #32157, 1000.000000000000114 ) ;
#6928=EDGE_CURVE ( 'NONE', #43155, #24145, #16474, .T. ) ;
#6929=ORIENTED_EDGE ( 'NONE', *, *, #43129, .F. ) ;
#6953=LINE ( 'NONE', #22603, #43922 ) ;
#6963=CARTESIAN_POINT ( 'NONE',  ( -215.0000000000000568, 164.9999999999999716, 111.9999999999999858 ) ) ;
#6964=DIRECTION ( 'NONE',  ( 0.8962124318248270161, -0.000000000000000000, 0.4436251537532894806 ) ) ;
#6965=CARTESIAN_POINT ( 'NONE',  ( -225.0000000000000568, 164.9999999999999716, 498.0000000000001137 ) ) ;
#6974=DIRECTION ( 'NONE',  ( 1.000000000000000000, -0.000000000000000000, -0.000000000000000000 ) ) ;
#6981=CARTESIAN_POINT ( 'NONE',  ( -167.4999999999999432, -102.5000000000000142, 10.00000000000000000 ) ) ;
#6987=VECTOR ( 'NONE', #26855, 999.9999999999998863 ) ;
#7003=CARTESIAN_POINT ( 'NONE',  ( -215.0000000000000568, 164.9999999999999716, 252.0000000000000000 ) ) ;
#7006=ORIENTED_EDGE ( 'NONE', *, *, #48422, .F. ) ;
#7022=ORIENTED_EDGE ( 'NONE', *, *, #2380, .T. ) ;
#7059=VECTOR ( 'NONE', #43429, 1000.000000000000000 ) ;
#7094=ORIENTED_EDGE ( 'NONE', *, *, #15775, .F. ) ;
#7112=CARTESIAN_POINT ( 'NONE',  ( -225.0000000000000568, 175.0000000000000000, 0.000000000000000000 ) ) ;
#7130=DIRECTION ( 'NONE',  ( 0.000000000000000000, 1.000000000000000000, 0.000000000000000000 ) ) ;
#7131=EDGE_CURVE ( 'NONE', #2021, #1277, #1891, .T. ) ;
#7164=VECTOR ( 'NONE', #47655, 1000.000000000000000 ) ;
#7179=ADVANCED_FACE ( 'NONE', ( #29340 ), #44949, .F. ) ;
#7183=ADVANCED_FACE ( 'NONE', ( #10089 ), #25746, .F. ) ;
#7257=DIRECTION ( 'NONE',  ( 0.000000000000000000, 1.000000000000000000, -1.604368532695312981E-16 ) ) ;
#7263=ORIENTED_EDGE ( 'NONE', *, *, #37324, .F. ) ;
#7288=CARTESIAN_POINT ( 'NONE',  ( -194.9999999999999432, 173.0000000000000000, 112.0000000000000000 ) ) ;
#7297=LINE ( 'NONE', #7562, #14293 ) ;
#7298=AXIS2_PLACEMENT_3D ( 'NONE', #29946, #45562, #18629 ) ;
#7308=DIRECTION ( 'NONE',  ( -1.000000000000000000, 0.000000000000000000, 0.000000000000000000 ) ) ;
#7336=AXIS2_PLACEMENT_3D ( 'NONE', #46828, #39694, #43771 ) ;
#7351=DIRECTION ( 'NONE',  ( 0.000000000000000000, 0.000000000000000000, -1.000000000000000000 ) ) ;
#7418=CARTESIAN_POINT ( 'NONE',  ( -50.00000000000000000, -50.00000000000000000, 900.0000000000000000 ) ) ;
#7439=CARTESIAN_POINT ( 'NONE',  ( -194.9999999999999432, -173.0000000000000000, 352.0000000000000568 ) ) ;
#7474=LINE ( 'NONE', #30063, #40687 ) ;
#7475=DIRECTION ( 'NONE',  ( 0.000000000000000000, 0.000000000000000000, 1.000000000000000000 ) ) ;
#7499=EDGE_LOOP ( 'NONE', ( #16944, #2537, #49672, #22984 ) ) ;
#7525=DIRECTION ( 'NONE',  ( -0.000000000000000000, -0.000000000000000000, 1.000000000000000000 ) ) ;
#7532=DIRECTION ( 'NONE',  ( 0.000000000000000000, 0.000000000000000000, -1.000000000000000000 ) ) ;
#7552=DIRECTION ( 'NONE',  ( 0.000000000000000000, -8.021842663476564905E-17, -1.000000000000000000 ) ) ;
#7554=PLANE ( 'NONE',  #21738 ) ;
#7562=CARTESIAN_POINT ( 'NONE',  ( -50.00000000000000000, -50.00000000000000000, 800.0000000000000000 ) ) ;
#7595=VECTOR ( 'NONE', #39885, 1000.000000000000000 ) ;
#7612=DIRECTION ( 'NONE',  ( -0.000000000000000000, -0.000000000000000000, 1.000000000000000000 ) ) ;
#7646=ORIENTED_EDGE ( 'NONE', *, *, #11085, .T. ) ;
#7667=ORIENTED_EDGE ( 'NONE', *, *, #25355, .T. ) ;
#7681=DIRECTION ( 'NONE',  ( 0.000000000000000000, 1.000000000000000000, 0.000000000000000000 ) ) ;
#7712=DIRECTION ( 'NONE',  ( 1.000000000000000000, 0.000000000000000000, -0.000000000000000000 ) ) ;
#7717=DIRECTION ( 'NONE',  ( 0.000000000000000000, 0.000000000000000000, -1.000000000000000000 ) ) ;
#7751=ORIENTED_EDGE ( 'NONE', *, *, #16405, .T. ) ;
#7781=CARTESIAN_POINT ( 'NONE',  ( 236.0000000000000000, -169.9999999999999716, 474.9999999999998863 ) ) ;
#7788=VECTOR ( 'NONE', #17316, 1000.000000000000000 ) ;
#7792=DIRECTION ( 'NONE',  ( -0.5038710255240859137, 0.000000000000000000, 0.8637789008984335659 ) ) ;
#7804=CARTESIAN_POINT ( 'NONE',  ( 167.4999999999999716, 74.83106485270648989, -120.5992382549688955 ) ) ;
#7813=DIRECTION ( 'NONE',  ( 0.000000000000000000, 0.000000000000000000, 1.000000000000000000 ) ) ;
#7819=ORIENTED_EDGE ( 'NONE', *, *, #6376, .F. ) ;
#7824=VECTOR ( 'NONE', #40859, 1000.000000000000000 ) ;
#7843=VERTEX_POINT ( 'NONE', #38128 ) ;
#7858=AXIS2_PLACEMENT_3D ( 'NONE', #38106, #21939, #37606 ) ;
#7864=CARTESIAN_POINT ( 'NONE',  ( 194.9999999999999716, 164.9999999999999716, 252.0000000000000000 ) ) ;
#7872=DIRECTION ( 'NONE',  ( -1.000000000000000000, 0.000000000000000000, -0.000000000000000000 ) ) ;
#7880=EDGE_LOOP ( 'NONE', ( #2585, #42701, #15661, #2157 ) ) ;
#7894=VERTEX_POINT ( 'NONE', #10650 ) ;
#7901=DIRECTION ( 'NONE',  ( 0.000000000000000000, -1.000000000000000000, 8.021842663476564905E-17 ) ) ;
#7914=VECTOR ( 'NONE', #50397, 1000.000000000000000 ) ;
#7943=LINE ( 'NONE', #46389, #47847 ) ;
#7954=ORIENTED_EDGE ( 'NONE', *, *, #13638, .F. ) ;
#7956=FACE_OUTER_BOUND ( 'NONE', #5618, .T. ) ;
#7970=ORIENTED_EDGE ( 'NONE', *, *, #31606, .F. ) ;
#7973=FACE_OUTER_BOUND ( 'NONE', #1830, .T. ) ;
#7984=LINE ( 'NONE', #47184, #47201 ) ;
#7986=ORIENTED_EDGE ( 'NONE', *, *, #50225, .F. ) ;
#8036=ORIENTED_EDGE ( 'NONE', *, *, #12499, .T. ) ;
#8054=VECTOR ( 'NONE', #44551, 1000.000000000000000 ) ;
#8061=EDGE_LOOP ( 'NONE', ( #11844, #40146, #23727, #25445 ) ) ;
#8067=ADVANCED_FACE ( 'NONE', ( #3448 ), #12922, .F. ) ;
#8089=ORIENTED_EDGE ( 'NONE', *, *, #1664, .F. ) ;
#8095=ORIENTED_EDGE ( 'NONE', *, *, #40998, .T. ) ;
#8117=ORIENTED_EDGE ( 'NONE', *, *, #9951, .F. ) ;
#8118=EDGE_CURVE ( 'NONE', #27665, #20648, #36054, .T. ) ;
#8124=LINE ( 'NONE', #39180, #48541 ) ;
#8150=ORIENTED_EDGE ( 'NONE', *, *, #26022, .F. ) ;
#8171=ORIENTED_EDGE ( 'NONE', *, *, #21153, .T. ) ;
#8175=LINE ( 'NONE', #4806, #25023 ) ;
#8188=CARTESIAN_POINT ( 'NONE',  ( -225.0000000000000568, 164.9999999999999716, 132.0000000000000000 ) ) ;
#8222=DIRECTION ( 'NONE',  ( -0.000000000000000000, -1.000000000000000000, -0.000000000000000000 ) ) ;
#8253=LINE ( 'NONE', #40066, #20633 ) ;
#8254=EDGE_CURVE ( 'NONE', #10051, #10114, #26008, .T. ) ;
#8274=ORIENTED_EDGE ( 'NONE', *, *, #33734, .F. ) ;
#8285=ORIENTED_EDGE ( 'NONE', *, *, #5152, .F. ) ;
#8296=VERTEX_POINT ( 'NONE', #7003 ) ;
#8301=EDGE_CURVE ( 'NONE', #41260, #17360, #9836, .T. ) ;
#8313=AXIS2_PLACEMENT_3D ( 'NONE', #386, #31696, #7308 ) ;
#8320=FACE_OUTER_BOUND ( 'NONE', #3034, .T. ) ;
#8333=FACE_OUTER_BOUND ( 'NONE', #20543, .T. ) ;
#8335=ORIENTED_EDGE ( 'NONE', *, *, #41760, .T. ) ;
#8377=PLANE ( 'NONE',  #968 ) ;
#8384=LINE ( 'NONE', #43261, #46105 ) ;
#8401=ADVANCED_FACE ( 'NONE', ( #11108 ), #27532, .F. ) ;
#8442=VECTOR ( 'NONE', #11219, 1000.000000000000000 ) ;
#8466=EDGE_LOOP ( 'NONE', ( #37845, #32161, #6115, #21510 ) ) ;
#8519=ORIENTED_EDGE ( 'NONE', *, *, #6765, .T. ) ;
#8534=LINE ( 'NONE', #39847, #16691 ) ;
#8547=ORIENTED_EDGE ( 'NONE', *, *, #24632, .T. ) ;
#8554=DIRECTION ( 'NONE',  ( -1.000000000000000000, 0.000000000000000000, 0.000000000000000000 ) ) ;
#8559=CARTESIAN_POINT ( 'NONE',  ( -0.5000000000000000000, -0.5000000000000000000, 1000.000000000000000 ) ) ;
#8564=CARTESIAN_POINT ( 'NONE',  ( 240.0000000000000000, -164.9999999999999716, 474.9999999999998863 ) ) ;
#8579=VECTOR ( 'NONE', #44415, 1000.000000000000000 ) ;
#8589=CARTESIAN_POINT ( 'NONE',  ( 194.9999999999999432, 173.0000000000000000, 352.0000000000000000 ) ) ;
#8632=EDGE_CURVE ( 'NONE', #11677, #1108, #14389, .T. ) ;
#8641=AXIS2_PLACEMENT_3D ( 'NONE', #21359, #32940, #9808 ) ;
#8650=ADVANCED_FACE ( 'NONE', ( #45657 ), #17481, .T. ) ;
#8689=CARTESIAN_POINT ( 'NONE',  ( -568.6915979970481203, 47.50000000000000000, -173.6700166912652890 ) ) ;
#8693=EDGE_CURVE ( 'NONE', #22974, #35388, #13861, .T. ) ;
#8701=LINE ( 'NONE', #32301, #44886 ) ;
#8748=LINE ( 'NONE', #32603, #38572 ) ;
#8750=EDGE_CURVE ( 'NONE', #33652, #40759, #18722, .T. ) ;
#8765=CARTESIAN_POINT ( 'NONE',  ( 214.9999999999999432, -175.0000000000000000, 10.00000000000000000 ) ) ;
#8769=EDGE_CURVE ( 'NONE', #9583, #8296, #27209, .T. ) ;
#8822=LINE ( 'NONE', #36032, #6096 ) ;
#8837=CARTESIAN_POINT ( 'NONE',  ( -177.4999999999999716, 112.5000000000000000, -10.00000000000000178 ) ) ;
#8864=ORIENTED_EDGE ( 'NONE', *, *, #2475, .T. ) ;
#8874=EDGE_CURVE ( 'NONE', #3623, #44566, #28476, .T. ) ;
#8903=FACE_OUTER_BOUND ( 'NONE', #49303, .T. ) ;
#8913=ORIENTED_EDGE ( 'NONE', *, *, #10025, .F. ) ;
#8928=VECTOR ( 'NONE', #39085, 1000.000000000000000 ) ;
#8965=ADVANCED_FACE ( 'NONE', ( #37451 ), #17907, .F. ) ;
#8986=VERTEX_POINT ( 'NONE', #49432 ) ;
#8989=AXIS2_PLACEMENT_3D ( 'NONE', #12054, #11290, #31566 ) ;
#9008=VERTEX_POINT ( 'NONE', #22526 ) ;
#9012=CARTESIAN_POINT ( 'NONE',  ( -178.1763882397827672, -62.49999999999998579, -120.5992382549688529 ) ) ;
#9022=VECTOR ( 'NONE', #9407, 1000.000000000000000 ) ;
#9024=VECTOR ( 'NONE', #29222, 1000.000000000000000 ) ;
#9042=EDGE_CURVE ( 'NONE', #9839, #835, #47300, .T. ) ;
#9060=CARTESIAN_POINT ( 'NONE',  ( 167.4999999999999716, 102.9547873477646647, -7.018571579996165433 ) ) ;
#9073=ORIENTED_EDGE ( 'NONE', *, *, #42945, .T. ) ;
#9193=CARTESIAN_POINT ( 'NONE',  ( 232.4999999999999716, -169.9999999999999716, 32.29650858650035161 ) ) ;
#9221=CARTESIAN_POINT ( 'NONE',  ( -194.9999999999999432, -173.0000000000000000, 352.0000000000000568 ) ) ;
#9223=VERTEX_POINT ( 'NONE', #25540 ) ;
#9226=ORIENTED_EDGE ( 'NONE', *, *, #26386, .T. ) ;
#9227=VECTOR ( 'NONE', #14477, 1000.000000000000000 ) ;
#9259=ADVANCED_FACE ( 'NONE', ( #38826 ), #43164, .F. ) ;
#9265=ORIENTED_EDGE ( 'NONE', *, *, #486, .T. ) ;
#9273=EDGE_CURVE ( 'NONE', #43883, #22983, #23915, .T. ) ;
#9288=ORIENTED_EDGE ( 'NONE', *, *, #31216, .F. ) ;
#9341=VECTOR ( 'NONE', #15656, 1000.000000000000000 ) ;
#9371=PLANE ( 'NONE',  #17504 ) ;
#9374=ADVANCED_FACE ( 'NONE', ( #35750 ), #582, .T. ) ;
#9381=DIRECTION ( 'NONE',  ( 0.000000000000000000, 0.000000000000000000, 1.000000000000000000 ) ) ;
#9407=DIRECTION ( 'NONE',  ( 0.000000000000000000, -1.000000000000000000, 0.000000000000000000 ) ) ;
#9430=PLANE ( 'NONE',  #32919 ) ;
#9447=DIRECTION ( 'NONE',  ( -1.000000000000000000, 0.000000000000000000, 0.000000000000000000 ) ) ;
#9467=CARTESIAN_POINT ( 'NONE',  ( 240.0000000000000000, -164.9999999999999716, 32.29650858650035161 ) ) ;
#9472=PLANE ( 'NONE',  #39582 ) ;
#9504=LINE ( 'NONE', #24917, #28269 ) ;
#9557=VECTOR ( 'NONE', #26538, 1000.000000000000000 ) ;
#9583=VERTEX_POINT ( 'NONE', #21571 ) ;
#9590=LINE ( 'NONE', #40888, #48345 ) ;
#9602=ORIENTED_EDGE ( 'NONE', *, *, #18181, .F. ) ;
#9633=CARTESIAN_POINT ( 'NONE',  ( 432.7825420346616170, 102.9547873477646647, -7.018571579996165433 ) ) ;
#9652=VERTEX_POINT ( 'NONE', #4548 ) ;
#9655=ADVANCED_FACE ( 'NONE', ( #24060 ), #43026, .F. ) ;
#9660=ORIENTED_EDGE ( 'NONE', *, *, #42903, .T. ) ;
#9673=VERTEX_POINT ( 'NONE', #27907 ) ;
#9680=CARTESIAN_POINT ( 'NONE',  ( 0.000000000000000000, -43.33333333333333570, 790.0000000000000000 ) ) ;
#9722=VERTEX_POINT ( 'NONE', #36120 ) ;
#9726=EDGE_LOOP ( 'NONE', ( #14547, #21611, #21138, #1675, #35607, #27449, #16566, #22388, #33800, #5390, #34985, #37680, #42247, #3860, #26715, #16156, #34500 ) ) ;
#9727=EDGE_LOOP ( 'NONE', ( #36338, #7751, #12589, #7986 ) ) ;
#9755=DIRECTION ( 'NONE',  ( -0.000000000000000000, -0.000000000000000000, -1.000000000000000000 ) ) ;
#9763=CARTESIAN_POINT ( 'NONE',  ( -567.5000000000000000, 57.49999999999996447, -183.5999999999997954 ) ) ;
#9773=DIRECTION ( 'NONE',  ( -1.000000000000000000, 0.000000000000000000, -0.000000000000000000 ) ) ;
#9808=DIRECTION ( 'NONE',  ( -1.000000000000000000, 0.000000000000000000, -0.000000000000000000 ) ) ;
#9814=CARTESIAN_POINT ( 'NONE',  ( 240.0000000000000000, -175.0000000000000000, 474.9999999999998863 ) ) ;
#9836=LINE ( 'NONE', #18277, #36051 ) ;
#9839=VERTEX_POINT ( 'NONE', #24553 ) ;
#9840=ORIENTED_EDGE ( 'NONE', *, *, #22462, .F. ) ;
#9856=CARTESIAN_POINT ( 'NONE',  ( 0.5000000000000000000, -0.5000000000000000000, 1000.000000000000000 ) ) ;
#9858=LINE ( 'NONE', #41155, #38034 ) ;
#9901=DIRECTION ( 'NONE',  ( -0.000000000000000000, -0.000000000000000000, -1.000000000000000000 ) ) ;
#9917=DIRECTION ( 'NONE',  ( -0.1191452206184309970, 0.000000000000000000, 0.9928768384869220975 ) ) ;
#9943=EDGE_CURVE ( 'NONE', #32080, #26268, #45531, .T. ) ;
#9951=EDGE_CURVE ( 'NONE', #46103, #11178, #23989, .T. ) ;
#9960=DIRECTION ( 'NONE',  ( 0.000000000000000000, -1.000000000000000000, 1.604368532695312981E-16 ) ) ;
#9964=LINE ( 'NONE', #28713, #12594 ) ;
#9970=CARTESIAN_POINT ( 'NONE',  ( -167.4999999999999432, -112.5000000000000000, -10.00000000000000000 ) ) ;
#9987=EDGE_LOOP ( 'NONE', ( #7263, #32871, #12133, #17955 ) ) ;
#9994=LINE ( 'NONE', #33608, #18028 ) ;
#10025=EDGE_CURVE ( 'NONE', #48660, #31445, #31189, .T. ) ;
#10045=DIRECTION ( 'NONE',  ( 0.000000000000000000, -0.4436251537532894806, 0.8962124318248270161 ) ) ;
#10051=VERTEX_POINT ( 'NONE', #39906 ) ;
#10089=FACE_OUTER_BOUND ( 'NONE', #12232, .T. ) ;
#10110=DIRECTION ( 'NONE',  ( -1.000000000000000000, 0.000000000000000000, 0.000000000000000000 ) ) ;
#10114=VERTEX_POINT ( 'NONE', #50626 ) ;
#10144=LINE ( 'NONE', #33762, #25478 ) ;
#10182=EDGE_CURVE ( 'NONE', #39878, #1277, #1153, .T. ) ;
#10191=CARTESIAN_POINT ( 'NONE',  ( 432.7825420346616170, -69.93075758371364259, -120.5992382549688671 ) ) ;
#10193=LINE ( 'NONE', #38668, #6987 ) ;
#10200=VECTOR ( 'NONE', #18824, 1000.000000000000114 ) ;
#10206=DIRECTION ( 'NONE',  ( 1.000000000000000000, -0.000000000000000000, -0.000000000000000000 ) ) ;
#10217=EDGE_CURVE ( 'NONE', #28864, #2021, #2399, .T. ) ;
#10220=DIRECTION ( 'NONE',  ( -0.000000000000000000, 0.000000000000000000, 1.000000000000000000 ) ) ;
#10246=CARTESIAN_POINT ( 'NONE',  ( -167.4999999999999716, -62.49999999999997158, -120.5992382549688671 ) ) ;
#10273=CARTESIAN_POINT ( 'NONE',  ( 194.9999999999999432, 164.9999999999999716, 112.0000000000000000 ) ) ;
#10277=CARTESIAN_POINT ( 'NONE',  ( -194.9999999999999432, 0.000000000000000000, 0.000000000000000000 ) ) ;
#10281=DIRECTION ( 'NONE',  ( 0.000000000000000000, 0.000000000000000000, -1.000000000000000000 ) ) ;
#10284=ORIENTED_EDGE ( 'NONE', *, *, #21486, .F. ) ;
#10305=ORIENTED_EDGE ( 'NONE', *, *, #18008, .F. ) ;
#10306=DIRECTION ( 'NONE',  ( 0.000000000000000000, 0.000000000000000000, -1.000000000000000000 ) ) ;
#10326=PLANE ( 'NONE',  #35446 ) ;
#10347=ORIENTED_EDGE ( 'NONE', *, *, #46797, .F. ) ;
#10351=VERTEX_POINT ( 'NONE', #28030 ) ;
#10366=ORIENTED_EDGE ( 'NONE', *, *, #39308, .F. ) ;
#10374=DIRECTION ( 'NONE',  ( 0.000000000000000000, 0.000000000000000000, 1.000000000000000000 ) ) ;
#10382=LINE ( 'NONE', #41673, #26403 ) ;
#10438=DIRECTION ( 'NONE',  ( -0.000000000000000000, -1.000000000000000000, -0.000000000000000000 ) ) ;
#10447=CARTESIAN_POINT ( 'NONE',  ( 232.4999999999999716, -169.9999999999999716, 4.999999999999616307 ) ) ;
#10450=AXIS2_PLACEMENT_3D ( 'NONE', #26601, #7612, #35340 ) ;
#10455=ADVANCED_FACE ( 'NONE', ( #31126 ), #341, .F. ) ;
#10457=DIRECTION ( 'NONE',  ( -1.000000000000000000, -0.000000000000000000, -0.000000000000000000 ) ) ;
#10461=EDGE_CURVE ( 'NONE', #42393, #47565, #43414, .T. ) ;
#10488=CARTESIAN_POINT ( 'NONE',  ( 177.5000000000000284, 112.5000000000000000, 0.000000000000000000 ) ) ;
#10517=VECTOR ( 'NONE', #45190, 1000.000000000000000 ) ;
#10606=CARTESIAN_POINT ( 'NONE',  ( -0.5000000000000000000, -0.5000000000000000000, 1000.000000000000000 ) ) ;
#10630=VECTOR ( 'NONE', #18087, 1000.000000000000000 ) ;
#10647=ORIENTED_EDGE ( 'NONE', *, *, #26581, .T. ) ;
#10650=CARTESIAN_POINT ( 'NONE',  ( 50.00000000000000000, 0.000000000000000000, 800.0000000000000000 ) ) ;
#10736=LINE ( 'NONE', #21793, #47487 ) ;
#10740=AXIS2_PLACEMENT_3D ( 'NONE', #19363, #15274, #38885 ) ;
#10742=ORIENTED_EDGE ( 'NONE', *, *, #38708, .F. ) ;
#10743=CARTESIAN_POINT ( 'NONE',  ( 236.0000000000000000, -169.9999999999999716, 62.29650858650038003 ) ) ;
#10746=CARTESIAN_POINT ( 'NONE',  ( -567.5000000000000000, 57.49999999999996447, -183.5999999999997954 ) ) ;
#10755=DIRECTION ( 'NONE',  ( -1.000000000000000000, 0.000000000000000000, 0.000000000000000000 ) ) ;
#10766=ORIENTED_EDGE ( 'NONE', *, *, #12405, .F. ) ;
#10795=PLANE ( 'NONE',  #11406 ) ;
#10811=ORIENTED_EDGE ( 'NONE', *, *, #40157, .T. ) ;
#10818=ORIENTED_EDGE ( 'NONE', *, *, #10217, .T. ) ;
#10821=CARTESIAN_POINT ( 'NONE',  ( -194.9999999999999432, 164.9999999999999716, 372.0000000000000000 ) ) ;
#10825=CARTESIAN_POINT ( 'NONE',  ( -582.5000000000000000, -72.50000000000001421, -58.60000000000003695 ) ) ;
#10838=VECTOR ( 'NONE', #48128, 1000.000000000000000 ) ;
#10862=VECTOR ( 'NONE', #7792, 1000.000000000000000 ) ;
#10868=ORIENTED_EDGE ( 'NONE', *, *, #38076, .F. ) ;
#10902=PLANE ( 'NONE',  #19673 ) ;
#10903=AXIS2_PLACEMENT_3D ( 'NONE', #27137, #35613, #42755 ) ;
#10905=CARTESIAN_POINT ( 'NONE',  ( 331.7552636306688214, 248.6897383013408387, 297.1446280767819985 ) ) ;
#10930=ORIENTED_EDGE ( 'NONE', *, *, #50551, .F. ) ;
#10944=VECTOR ( 'NONE', #49990, 1000.000000000000000 ) ;
#10953=VECTOR ( 'NONE', #40822, 1000.000000000000114 ) ;
#10979=DIRECTION ( 'NONE',  ( 0.000000000000000000, 0.000000000000000000, -1.000000000000000000 ) ) ;
#11003=CARTESIAN_POINT ( 'NONE',  ( 224.9999999999999716, 175.0000000000000284, 499.9999999999998863 ) ) ;
#11013=DIRECTION ( 'NONE',  ( 0.000000000000000000, -0.2981428420003837121, -0.9545212652235329776 ) ) ;
#11017=DIRECTION ( 'NONE',  ( 0.000000000000000000, -1.000000000000000000, 0.000000000000000000 ) ) ;
#11019=LINE ( 'NONE', #15386, #23888 ) ;
#11024=AXIS2_PLACEMENT_3D ( 'NONE', #1465, #9901, #48352 ) ;
#11031=DIRECTION ( 'NONE',  ( 0.000000000000000000, 1.000000000000000000, 0.000000000000000000 ) ) ;
#11047=DIRECTION ( 'NONE',  ( -1.000000000000000000, 0.000000000000000000, 0.000000000000000000 ) ) ;
#11048=ORIENTED_EDGE ( 'NONE', *, *, #16222, .F. ) ;
#11073=ADVANCED_FACE ( 'NONE', ( #22282 ), #45097, .F. ) ;
#11076=LINE ( 'NONE', #46185, #40616 ) ;
#11077=VECTOR ( 'NONE', #7901, 1000.000000000000000 ) ;
#11085=EDGE_CURVE ( 'NONE', #36453, #18948, #30232, .T. ) ;
#11087=DIRECTION ( 'NONE',  ( -1.000000000000000000, -8.881784197001252323E-16, 0.000000000000000000 ) ) ;
#11091=( GEOMETRIC_REPRESENTATION_CONTEXT ( 3 ) GLOBAL_UNCERTAINTY_ASSIGNED_CONTEXT ( ( #42900 ) ) GLOBAL_UNIT_ASSIGNED_CONTEXT ( ( #50597, #27566, #39371 ) ) REPRESENTATION_CONTEXT ( 'NONE', 'WORKASPACE' ) );
#11108=FACE_OUTER_BOUND ( 'NONE', #3778, .T. ) ;
#11113=ORIENTED_EDGE ( 'NONE', *, *, #8769, .T. ) ;
#11115=VECTOR ( 'NONE', #7257, 1000.000000000000000 ) ;
#11146=CARTESIAN_POINT ( 'NONE',  ( 194.9999999999999432, 173.0000000000000000, 231.9999999999999716 ) ) ;
#11147=ORIENTED_EDGE ( 'NONE', *, *, #22363, .T. ) ;
#11161=AXIS2_PLACEMENT_3D ( 'NONE', #1848, #21336, #10045 ) ;
#11165=VERTEX_POINT ( 'NONE', #31518 ) ;
#11178=VERTEX_POINT ( 'NONE', #19176 ) ;
#11179=ORIENTED_EDGE ( 'NONE', *, *, #39039, .F. ) ;
#11187=LINE ( 'NONE', #42217, #14097 ) ;
#11211=CARTESIAN_POINT ( 'NONE',  ( 0.000000000000000000, 0.000000000000000000, 900.0000000000000000 ) ) ;
#11215=VERTEX_POINT ( 'NONE', #20445 ) ;
#11219=DIRECTION ( 'NONE',  ( -1.000000000000000000, 0.000000000000000000, 0.000000000000000000 ) ) ;
#11225=CARTESIAN_POINT ( 'NONE',  ( -225.0000000000000568, 164.9999999999999716, 252.0000000000000000 ) ) ;
#11237=CARTESIAN_POINT ( 'NONE',  ( 194.9999999999999432, 173.0000000000000000, 112.0000000000000000 ) ) ;
#11257=DIRECTION ( 'NONE',  ( 1.000000000000000000, -0.000000000000000000, -0.000000000000000000 ) ) ;
#11290=DIRECTION ( 'NONE',  ( 1.000000000000000000, 0.000000000000000000, -0.000000000000000000 ) ) ;
#11315=CARTESIAN_POINT ( 'NONE',  ( 50.00000000000002132, 0.000000000000000000, 899.9999999999998863 ) ) ;
#11317=VERTEX_POINT ( 'NONE', #31771 ) ;
#11360=CARTESIAN_POINT ( 'NONE',  ( 177.5000000000000284, -112.5000000000000000, -10.00000000000000000 ) ) ;
#11361=DIRECTION ( 'NONE',  ( 0.000000000000000000, 1.000000000000000000, 0.000000000000000000 ) ) ;
#11378=ORIENTED_EDGE ( 'NONE', *, *, #23372, .F. ) ;
#11380=CARTESIAN_POINT ( 'NONE',  ( 7.884183412771418986, -42.26678417219199702, 893.0811050474360400 ) ) ;
#11388=DIRECTION ( 'NONE',  ( 0.000000000000000000, 1.604368532695312981E-16, 1.000000000000000000 ) ) ;
#11396=EDGE_LOOP ( 'NONE', ( #10647, #28454, #597, #50035 ) ) ;
#11402=AXIS2_PLACEMENT_3D ( 'NONE', #47459, #48214, #16964 ) ;
#11406=AXIS2_PLACEMENT_3D ( 'NONE', #45669, #42091, #26713 ) ;
#11432=ORIENTED_EDGE ( 'NONE', *, *, #47722, .T. ) ;
#11512=ORIENTED_EDGE ( 'NONE', *, *, #13177, .T. ) ;
#11515=CARTESIAN_POINT ( 'NONE',  ( 33.89193117067290473, 21.24469349090191983, 910.0000000000000000 ) ) ;
#11528=EDGE_CURVE ( 'NONE', #49308, #36027, #12380, .T. ) ;
#11541=EDGE_CURVE ( 'NONE', #16449, #24983, #42914, .T. ) ;
#11557=ORIENTED_EDGE ( 'NONE', *, *, #44926, .F. ) ;
#11563=DIRECTION ( 'NONE',  ( 0.000000000000000000, -1.000000000000000000, -0.000000000000000000 ) ) ;
#11578=FACE_OUTER_BOUND ( 'NONE', #39591, .T. ) ;
#11594=CARTESIAN_POINT ( 'NONE',  ( 50.00000000000000000, -50.00000000000000000, 900.0000000000000000 ) ) ;
#11605=ORIENTED_EDGE ( 'NONE', *, *, #48140, .F. ) ;
#11606=ORIENTED_EDGE ( 'NONE', *, *, #3581, .F. ) ;
#11640=EDGE_LOOP ( 'NONE', ( #18726, #26186, #37435, #3528 ) ) ;
#11648=VERTEX_POINT ( 'NONE', #48496 ) ;
#11649=PLANE ( 'NONE',  #46292 ) ;
#11653=FACE_BOUND ( 'NONE', #34978, .T. ) ;
#11668=PLANE ( 'NONE',  #10740 ) ;
#11677=VERTEX_POINT ( 'NONE', #44907 ) ;
#11687=AXIS2_PLACEMENT_3D ( 'NONE', #49725, #23591, #31309 ) ;
#11695=EDGE_LOOP ( 'NONE', ( #10868, #25158, #44901, #32406 ) ) ;
#11699=PLANE ( 'NONE',  #36378 ) ;
#11703=PLANE ( 'NONE',  #15167 ) ;
#11707=CARTESIAN_POINT ( 'NONE',  ( -194.9999999999999432, 164.9999999999999716, 500.0000000000000000 ) ) ;
#11708=CARTESIAN_POINT ( 'NONE',  ( 177.5000000000000000, -112.5000000000000000, -9.999999999999973355 ) ) ;
#11710=DIRECTION ( 'NONE',  ( -0.000000000000000000, -0.000000000000000000, -1.000000000000000000 ) ) ;
#11723=DIRECTION ( 'NONE',  ( 1.000000000000000000, 0.000000000000000000, 0.000000000000000000 ) ) ;
#11725=VECTOR ( 'NONE', #50156, 1000.000000000000000 ) ;
#11764=LINE ( 'NONE', #19452, #43867 ) ;
#11773=AXIS2_PLACEMENT_3D ( 'NONE', #16026, #31689, #4966 ) ;
#11793=ORIENTED_EDGE ( 'NONE', *, *, #39046, .T. ) ;
#11798=EDGE_CURVE ( 'NONE', #35326, #22662, #22345, .T. ) ;
#11811=ORIENTED_EDGE ( 'NONE', *, *, #19868, .T. ) ;
#11844=ORIENTED_EDGE ( 'NONE', *, *, #19842, .F. ) ;
#11871=CARTESIAN_POINT ( 'NONE',  ( 432.7825420346616170, -112.5000000000000000, -9.999999999999973355 ) ) ;
#11899=DIRECTION ( 'NONE',  ( 0.000000000000000000, 0.000000000000000000, 1.000000000000000000 ) ) ;
#11938=CARTESIAN_POINT ( 'NONE',  ( -177.4999999999999716, 57.49999999999996447, -130.5992382549688671 ) ) ;
#11959=FACE_OUTER_BOUND ( 'NONE', #4796, .T. ) ;
#11962=CARTESIAN_POINT ( 'NONE',  ( 214.9999999999999432, 164.9999999999999716, 372.0000000000000000 ) ) ;
#11975=AXIS2_PLACEMENT_3D ( 'NONE', #26024, #17308, #21920 ) ;
#11977=FACE_OUTER_BOUND ( 'NONE', #35206, .T. ) ;
#12023=DIRECTION ( 'NONE',  ( 1.000000000000000000, 0.000000000000000000, 0.000000000000000000 ) ) ;
#12054=CARTESIAN_POINT ( 'NONE',  ( -194.9999999999999432, 0.000000000000000000, 0.000000000000000000 ) ) ;
#12100=EDGE_CURVE ( 'NONE', #24711, #17183, #29241, .T. ) ;
#12127=DIRECTION ( 'NONE',  ( 0.000000000000000000, 0.2791762785758810650, -0.9602398687205827565 ) ) ;
#12133=ORIENTED_EDGE ( 'NONE', *, *, #3326, .T. ) ;
#12150=DIRECTION ( 'NONE',  ( 0.000000000000000000, 0.2981428420003837121, 0.9545212652235329776 ) ) ;
#12162=LINE ( 'NONE', #624, #7595 ) ;
#12164=VERTEX_POINT ( 'NONE', #10246 ) ;
#12172=CARTESIAN_POINT ( 'NONE',  ( -568.8466156985925863, 57.49999999999996447, -173.6910835022032700 ) ) ;
#12175=CARTESIAN_POINT ( 'NONE',  ( 228.9999999999999716, -169.9999999999999716, 4.999999999999616307 ) ) ;
#12190=LINE ( 'NONE', #20384, #41171 ) ;
#12210=FACE_OUTER_BOUND ( 'NONE', #45584, .T. ) ;
#12216=CIRCLE ( 'NONE', #29427, 3.500000000000003109 ) ;
#12221=VECTOR ( 'NONE', #21292, 1000.000000000000000 ) ;
#12232=EDGE_LOOP ( 'NONE', ( #21216, #4045, #23734, #22737 ) ) ;
#12252=EDGE_CURVE ( 'NONE', #23225, #27522, #10736, .T. ) ;
#12275=CARTESIAN_POINT ( 'NONE',  ( -582.5000000000000000, -72.50000000000001421, -58.60000000000003695 ) ) ;
#12293=ORIENTED_EDGE ( 'NONE', *, *, #44640, .F. ) ;
#12295=LINE ( 'NONE', #19997, #15822 ) ;
#12312=VECTOR ( 'NONE', #26756, 1000.000000000000114 ) ;
#12338=ORIENTED_EDGE ( 'NONE', *, *, #5109, .T. ) ;
#12341=LINE ( 'NONE', #23900, #26968 ) ;
#12353=LINE ( 'NONE', #4671, #40514 ) ;
#12354=MECHANICAL_DESIGN_GEOMETRIC_PRESENTATION_REPRESENTATION('',(#22971),#27086);
#12380=LINE ( 'NONE', #20082, #40739 ) ;
#12388=EDGE_LOOP ( 'NONE', ( #6409, #6274, #42966 ) ) ;
#12405=EDGE_CURVE ( 'NONE', #39651, #11178, #43302, .T. ) ;
#12412=DIRECTION ( 'NONE',  ( 0.000000000000000000, 0.000000000000000000, -1.000000000000000000 ) ) ;
#12413=DIRECTION ( 'NONE',  ( -0.9908916497796512735, 0.000000000000000000, -0.1346615698592613652 ) ) ;
#12423=DIRECTION ( 'NONE',  ( 0.000000000000000000, -1.000000000000000000, 1.604368532695312981E-16 ) ) ;
#12451=VECTOR ( 'NONE', #18746, 1000.000000000000000 ) ;
#12455=VERTEX_POINT ( 'NONE', #5319 ) ;
#12462=AXIS2_PLACEMENT_3D ( 'NONE', #6025, #22193, #6789 ) ;
#12481=AXIS2_PLACEMENT_3D ( 'NONE', #15429, #31086, #14922 ) ;
#12499=EDGE_CURVE ( 'NONE', #31445, #4257, #44054, .T. ) ;
#12517=FACE_OUTER_BOUND ( 'NONE', #48961, .T. ) ;
#12535=DIRECTION ( 'NONE',  ( 0.000000000000000000, 0.000000000000000000, -1.000000000000000000 ) ) ;
#12559=ORIENTED_EDGE ( 'NONE', *, *, #22229, .F. ) ;
#12582=PRODUCT_CONTEXT ( 'NONE', #1417, 'mechanical' ) ;
#12584=CARTESIAN_POINT ( 'NONE',  ( 0.000000000000000000, 0.000000000000000000, 10.00000000000000000 ) ) ;
#12589=ORIENTED_EDGE ( 'NONE', *, *, #15157, .F. ) ;
#12594=VECTOR ( 'NONE', #10220, 1000.000000000000000 ) ;
#12601=CARTESIAN_POINT ( 'NONE',  ( -194.9999999999999432, 173.0000000000000000, 132.0000000000000000 ) ) ;
#12608=VECTOR ( 'NONE', #11710, 1000.000000000000000 ) ;
#12638=CARTESIAN_POINT ( 'NONE',  ( 177.5000000000000284, -112.5000000000000000, -10.00000000000000000 ) ) ;
#12694=AXIS2_PLACEMENT_3D ( 'NONE', #46196, #22885, #3123 ) ;
#12703=ORIENTED_EDGE ( 'NONE', *, *, #40307, .T. ) ;
#12708=ORIENTED_EDGE ( 'NONE', *, *, #25844, .F. ) ;
#12716=EDGE_CURVE ( 'NONE', #835, #44977, #31462, .T. ) ;
#12724=AXIS2_PLACEMENT_3D ( 'NONE', #337, #47733, #47486 ) ;
#12746=VERTEX_POINT ( 'NONE', #11962 ) ;
#12776=VECTOR ( 'NONE', #49440, 1000.000000000000000 ) ;
#12785=CARTESIAN_POINT ( 'NONE',  ( -177.4999999999999716, 57.49999999999996447, -9.999999999999973355 ) ) ;
#12829=DIRECTION ( 'NONE',  ( 0.000000000000000000, 0.000000000000000000, 1.000000000000000000 ) ) ;
#12838=ORIENTED_EDGE ( 'NONE', *, *, #44460, .T. ) ;
#12860=EDGE_LOOP ( 'NONE', ( #35370, #8864, #40956, #45795, #19166 ) ) ;
#12870=VECTOR ( 'NONE', #47632, 1000.000000000000000 ) ;
#12891=VERTEX_POINT ( 'NONE', #47313 ) ;
#12895=CARTESIAN_POINT ( 'NONE',  ( -1.387778780781445676E-14, -6.938893903907228378E-14, 978.4685478195414134 ) ) ;
#12914=ORIENTED_EDGE ( 'NONE', *, *, #37121, .F. ) ;
#12922=PLANE ( 'NONE',  #16360 ) ;
#12958=DIRECTION ( 'NONE',  ( 0.000000000000000000, 0.9545212652235329776, -0.2981428420003837121 ) ) ;
#12971=AXIS2_PLACEMENT_3D ( 'NONE', #5951, #29310, #49514 ) ;
#13035=PRODUCT_DEFINITION ( 'UNKNOWN', '', #37356, #39611 ) ;
#13045=CARTESIAN_POINT ( 'NONE',  ( 177.5000000000000284, -112.5000000000000000, 0.000000000000000000 ) ) ;
#13081=DIRECTION ( 'NONE',  ( 1.000000000000000000, -0.000000000000000000, 0.000000000000000000 ) ) ;
#13082=EDGE_CURVE ( 'NONE', #30057, #46103, #40008, .T. ) ;
#13151=CARTESIAN_POINT ( 'NONE',  ( -50.00000000000000000, -50.00000000000000000, 800.0000000000000000 ) ) ;
#13157=ORIENTED_EDGE ( 'NONE', *, *, #36523, .F. ) ;
#13163=LINE ( 'NONE', #20611, #34029 ) ;
#13165=LINE ( 'NONE', #37051, #43652 ) ;
#13169=DIRECTION ( 'NONE',  ( 0.5038710255240862468, 0.000000000000000000, 0.8637789008984334549 ) ) ;
#13177=EDGE_CURVE ( 'NONE', #15989, #36849, #47387, .T. ) ;
#13178=CARTESIAN_POINT ( 'NONE',  ( 0.000000000000000000, -49.99999999999994316, 800.0000000000001137 ) ) ;
#13201=LINE ( 'NONE', #28858, #31657 ) ;
#13209=ORIENTED_EDGE ( 'NONE', *, *, #38112, .F. ) ;
#13220=ORIENTED_EDGE ( 'NONE', *, *, #18938, .F. ) ;
#13227=CARTESIAN_POINT ( 'NONE',  ( 214.9999999999999432, -175.0000000000000000, 497.2965085865001811 ) ) ;
#13249=CARTESIAN_POINT ( 'NONE',  ( -225.0000000000000568, -165.6999999999999602, 254.8599999999999852 ) ) ;
#13265=DIRECTION ( 'NONE',  ( 1.000000000000000000, 0.000000000000000000, 0.000000000000000000 ) ) ;
#13283=EDGE_CURVE ( 'NONE', #41907, #16490, #37180, .T. ) ;
#13293=EDGE_LOOP ( 'NONE', ( #32537, #9073, #1670 ) ) ;
#13296=CARTESIAN_POINT ( 'NONE',  ( 214.9999999999999432, 173.0000000000000000, 352.0000000000000000 ) ) ;
#13313=EDGE_CURVE ( 'NONE', #50400, #7894, #23724, .T. ) ;
#13318=EDGE_CURVE ( 'NONE', #6437, #15488, #48645, .T. ) ;
#13327=ORIENTED_EDGE ( 'NONE', *, *, #18324, .F. ) ;
#13366=VECTOR ( 'NONE', #41953, 1000.000000000000000 ) ;
#13368=EDGE_CURVE ( 'NONE', #4257, #8296, #39192, .T. ) ;
#13388=DIRECTION ( 'NONE',  ( -0.000000000000000000, -0.000000000000000000, -1.000000000000000000 ) ) ;
#13389=CARTESIAN_POINT ( 'NONE',  ( -194.9999999999999432, 173.0000000000000000, 132.0000000000000000 ) ) ;
#13416=EDGE_CURVE ( 'NONE', #13689, #31054, #22051, .T. ) ;
#13433=VECTOR ( 'NONE', #31325, 1000.000000000000000 ) ;
#13458=ORIENTED_EDGE ( 'NONE', *, *, #1101, .F. ) ;
#13461=LINE ( 'NONE', #31975, #42892 ) ;
#13463=ORIENTED_EDGE ( 'NONE', *, *, #43129, .T. ) ;
#13464=EDGE_CURVE ( 'NONE', #43486, #48005, #4041, .T. ) ;
#13478=DIRECTION ( 'NONE',  ( 1.000000000000000000, 0.000000000000000000, 0.000000000000000000 ) ) ;
#13489=CIRCLE ( 'NONE', #15961, 40.00000000000000000 ) ;
#13529=DIRECTION ( 'NONE',  ( -0.000000000000000000, 1.000000000000000000, -2.406552799042969348E-16 ) ) ;
#13573=EDGE_LOOP ( 'NONE', ( #7006, #42644, #45732, #25475, #44998, #23480, #39214, #16931 ) ) ;
#13574=CARTESIAN_POINT ( 'NONE',  ( 0.000000000000000000, 326.6272189349111841, 136.0946745562129649 ) ) ;
#13585=ADVANCED_FACE ( 'NONE', ( #15824 ), #5022, .T. ) ;
#13604=VERTEX_POINT ( 'NONE', #187 ) ;
#13610=VERTEX_POINT ( 'NONE', #47077 ) ;
#13628=CARTESIAN_POINT ( 'NONE',  ( 0.000000000000000000, -397.9839762253770346, 197.0020682315616796 ) ) ;
#13638=EDGE_CURVE ( 'NONE', #48180, #43354, #33760, .T. ) ;
#13689=VERTEX_POINT ( 'NONE', #21684 ) ;
#13726=FACE_OUTER_BOUND ( 'NONE', #2817, .T. ) ;
#13758=EDGE_CURVE ( 'NONE', #24673, #9673, #15698, .T. ) ;
#13759=CARTESIAN_POINT ( 'NONE',  ( 33.89193117067290473, -21.24469349090191983, 910.0000000000000000 ) ) ;
#13803=CARTESIAN_POINT ( 'NONE',  ( -194.9999999999999432, -172.9999999999999716, 232.0000000000000284 ) ) ;
#13806=DIRECTION ( 'NONE',  ( -0.000000000000000000, 0.000000000000000000, 1.000000000000000000 ) ) ;
#13816=ORIENTED_EDGE ( 'NONE', *, *, #9951, .T. ) ;
#13830=CARTESIAN_POINT ( 'NONE',  ( 214.9999999999999432, 164.9999999999999716, 500.0000000000000000 ) ) ;
#13838=AXIS2_PLACEMENT_3D ( 'NONE', #44931, #33931, #25469 ) ;
#13849=ORIENTED_EDGE ( 'NONE', *, *, #26524, .F. ) ;
#13861=LINE ( 'NONE', #38273, #22945 ) ;
#13863=PLANE ( 'NONE',  #25749 ) ;
#13869=AXIS2_PLACEMENT_3D ( 'NONE', #12601, #24674, #17222 ) ;
#13897=ADVANCED_FACE ( 'NONE', ( #29020 ), #33143, .T. ) ;
#13911=ORIENTED_EDGE ( 'NONE', *, *, #43711, .T. ) ;
#13918=EDGE_CURVE ( 'NONE', #43354, #12746, #16971, .T. ) ;
#13919=DIRECTION ( 'NONE',  ( -1.000000000000000000, 0.000000000000000000, 0.000000000000000000 ) ) ;
#13921=VECTOR ( 'NONE', #31063, 1000.000000000000000 ) ;
#13954=VECTOR ( 'NONE', #1239, 1000.000000000000000 ) ;
#13964=ORIENTED_EDGE ( 'NONE', *, *, #31285, .T. ) ;
#13984=DIRECTION ( 'NONE',  ( -0.000000000000000000, -1.000000000000000000, -0.000000000000000000 ) ) ;
#13987=EDGE_CURVE ( 'NONE', #30057, #39651, #29775, .T. ) ;
#13988=DIRECTION ( 'NONE',  ( 0.000000000000000000, -0.000000000000000000, 1.000000000000000000 ) ) ;
#14029=CARTESIAN_POINT ( 'NONE',  ( 432.7825420346616170, 67.47808924524053964, -120.5992382549688955 ) ) ;
#14039=ORIENTED_EDGE ( 'NONE', *, *, #13416, .T. ) ;
#14041=ADVANCED_FACE ( 'NONE', ( #33636 ), #45393, .T. ) ;
#14056=EDGE_CURVE ( 'NONE', #42074, #33060, #43331, .T. ) ;
#14070=ORIENTED_EDGE ( 'NONE', *, *, #32846, .T. ) ;
#14093=ADVANCED_FACE ( 'NONE', ( #7956 ), #31312, .T. ) ;
#14097=VECTOR ( 'NONE', #23741, 1000.000000000000000 ) ;
#14100=VERTEX_POINT ( 'NONE', #23854 ) ;
#14146=AXIS2_PLACEMENT_3D ( 'NONE', #1598, #40836, #17246 ) ;
#14149=LINE ( 'NONE', #17513, #19253 ) ;
#14208=EDGE_CURVE ( 'NONE', #25022, #44965, #1514, .T. ) ;
#14246=ORIENTED_EDGE ( 'NONE', *, *, #30501, .T. ) ;
#14249=DIRECTION ( 'NONE',  ( 0.4055129968046615185, -0.4055129968046615185, -0.8192181753629523833 ) ) ;
#14293=VECTOR ( 'NONE', #37610, 1000.000000000000000 ) ;
#14331=LINE ( 'NONE', #10488, #45761 ) ;
#14354=ORIENTED_EDGE ( 'NONE', *, *, #29081, .F. ) ;
#14359=DIRECTION ( 'NONE',  ( 0.000000000000000000, 1.000000000000000000, -1.822804496942679766E-16 ) ) ;
#14376=ORIENTED_EDGE ( 'NONE', *, *, #35896, .T. ) ;
#14379=AXIS2_PLACEMENT_3D ( 'NONE', #5645, #28756, #21300 ) ;
#14384=ORIENTED_EDGE ( 'NONE', *, *, #16984, .T. ) ;
#14385=CARTESIAN_POINT ( 'NONE',  ( -215.0000000000000568, 164.9999999999999716, 372.0000000000000000 ) ) ;
#14388=AXIS2_PLACEMENT_3D ( 'NONE', #34552, #6076, #14528 ) ;
#14389=LINE ( 'NONE', #21848, #45831 ) ;
#14433=PLANE ( 'NONE',  #12694 ) ;
#14442=VERTEX_POINT ( 'NONE', #43015 ) ;
#14452=EDGE_LOOP ( 'NONE', ( #14376, #34470, #16769, #34411 ) ) ;
#14461=AXIS2_PLACEMENT_3D ( 'NONE', #1251, #21734, #33310 ) ;
#14465=AXIS2_PLACEMENT_3D ( 'NONE', #3398, #594, #46725 ) ;
#14468=VERTEX_POINT ( 'NONE', #19425 ) ;
#14477=DIRECTION ( 'NONE',  ( -0.000000000000000000, 1.000000000000000000, -1.604368532695312981E-16 ) ) ;
#14496=PLANE ( 'NONE',  #41043 ) ;
#14528=DIRECTION ( 'NONE',  ( 0.000000000000000000, 0.000000000000000000, -1.000000000000000000 ) ) ;
#14547=ORIENTED_EDGE ( 'NONE', *, *, #49914, .F. ) ;
#14559=DIRECTION ( 'NONE',  ( 0.000000000000000000, -1.000000000000000000, 0.000000000000000000 ) ) ;
#14572=FACE_OUTER_BOUND ( 'NONE', #42537, .T. ) ;
#14585=LINE ( 'NONE', #38711, #6494 ) ;
#14622=DIRECTION ( 'NONE',  ( 0.000000000000000000, -1.000000000000000000, 0.000000000000000000 ) ) ;
#14651=EDGE_CURVE ( 'NONE', #4161, #15488, #33012, .T. ) ;
#14669=VECTOR ( 'NONE', #23027, 1000.000000000000000 ) ;
#14706=EDGE_CURVE ( 'NONE', #44330, #16449, #29394, .T. ) ;
#14712=LINE ( 'NONE', #45976, #10862 ) ;
#14746=ADVANCED_FACE ( 'NONE', ( #41954 ), #10902, .F. ) ;
#14747=VECTOR ( 'NONE', #20007, 1000.000000000000000 ) ;
#14748=DIRECTION ( 'NONE',  ( 0.000000000000000000, -1.000000000000000000, 1.604368532695312981E-16 ) ) ;
#14751=DIRECTION ( 'NONE',  ( 0.000000000000000000, 0.000000000000000000, -1.000000000000000000 ) ) ;
#14753=CARTESIAN_POINT ( 'NONE',  ( -225.0000000000000568, 164.9999999999999716, 111.9999999999999858 ) ) ;
#14760=VECTOR ( 'NONE', #45599, 1000.000000000000000 ) ;
#14763=VECTOR ( 'NONE', #43966, 1000.000000000000000 ) ;
#14773=ADVANCED_FACE ( 'NONE', ( #38631, #38376 ), #15518, .T. ) ;
#14784=VERTEX_POINT ( 'NONE', #31183 ) ;
#14792=DIRECTION ( 'NONE',  ( -1.000000000000000000, -0.000000000000000000, -0.000000000000000000 ) ) ;
#14803=VECTOR ( 'NONE', #33573, 1000.000000000000000 ) ;
#14811=ORIENTED_EDGE ( 'NONE', *, *, #37188, .T. ) ;
#14818=LINE ( 'NONE', #42016, #20892 ) ;
#14839=CARTESIAN_POINT ( 'NONE',  ( -167.4999999999999432, -112.5000000000000000, 10.00000000000000000 ) ) ;
#14863=ORIENTED_EDGE ( 'NONE', *, *, #44461, .T. ) ;
#14888=EDGE_CURVE ( 'NONE', #5210, #11165, #24750, .T. ) ;
#14893=CARTESIAN_POINT ( 'NONE',  ( 214.9999999999999432, -172.9999999999999716, 232.0000000000000284 ) ) ;
#14917=VECTOR ( 'NONE', #46192, 1000.000000000000000 ) ;
#14922=DIRECTION ( 'NONE',  ( -1.000000000000000000, 0.000000000000000000, 0.000000000000000000 ) ) ;
#14934=EDGE_CURVE ( 'NONE', #20787, #19082, #44712, .T. ) ;
#14944=DIRECTION ( 'NONE',  ( -1.000000000000000000, 0.000000000000000000, 0.000000000000000000 ) ) ;
#14947=VECTOR ( 'NONE', #2667, 1000.000000000000000 ) ;
#14978=AXIS2_PLACEMENT_3D ( 'NONE', #22184, #25780, #30133 ) ;
#15032=CARTESIAN_POINT ( 'NONE',  ( 432.7825420346616170, -77.43746236555679729, -130.5992382549688671 ) ) ;
#15037=CARTESIAN_POINT ( 'NONE',  ( 33.89193117067290473, 21.24469349090191983, 910.0000000000000000 ) ) ;
#15042=CARTESIAN_POINT ( 'NONE',  ( -178.1763882397831082, 74.83106485270566566, -120.5992382549688955 ) ) ;
#15043=CARTESIAN_POINT ( 'NONE',  ( -239.0000000000000853, -153.6999999999999602, 254.8599999999999852 ) ) ;
#15055=CARTESIAN_POINT ( 'NONE',  ( 214.9999999999999432, 173.0000000000000000, 372.0000000000000000 ) ) ;
#15069=CARTESIAN_POINT ( 'NONE',  ( -568.6915979970481203, 57.49999999999996447, -173.6700166912652890 ) ) ;
#15074=DIRECTION ( 'NONE',  ( 0.000000000000000000, -0.2981428420003837121, -0.9545212652235329776 ) ) ;
#15115=FACE_OUTER_BOUND ( 'NONE', #47670, .T. ) ;
#15139=VERTEX_POINT ( 'NONE', #34729 ) ;
#15157=EDGE_CURVE ( 'NONE', #2566, #15989, #27269, .T. ) ;
#15167=AXIS2_PLACEMENT_3D ( 'NONE', #27357, #42993, #7872 ) ;
#15170=DIRECTION ( 'NONE',  ( -0.000000000000000000, -0.000000000000000000, 1.000000000000000000 ) ) ;
#15190=ORIENTED_EDGE ( 'NONE', *, *, #31343, .T. ) ;
#15196=EDGE_CURVE ( 'NONE', #35891, #9839, #31886, .T. ) ;
#15221=CARTESIAN_POINT ( 'NONE',  ( 0.000000000000000000, -164.9999999999999716, 0.000000000000000000 ) ) ;
#15225=ORIENTED_EDGE ( 'NONE', *, *, #5254, .T. ) ;
#15234=ORIENTED_EDGE ( 'NONE', *, *, #38076, .T. ) ;
#15254=SHAPE_REPRESENTATION_RELATIONSHIP ( 'NONE' , 'NONE' ,  #15926, #24018 ) ;
#15260=ORIENTED_EDGE ( 'NONE', *, *, #26518, .F. ) ;
#15264=LINE ( 'NONE', #15754, #22826 ) ;
#15274=DIRECTION ( 'NONE',  ( -0.8637789008984334549, 0.000000000000000000, 0.5038710255240862468 ) ) ;
#15278=EDGE_CURVE ( 'NONE', #16638, #11677, #40084, .T. ) ;
#15284=DIRECTION ( 'NONE',  ( 0.000000000000000000, 0.000000000000000000, 1.000000000000000000 ) ) ;
#15307=EDGE_LOOP ( 'NONE', ( #36680, #18248, #24798, #49353 ) ) ;
#15311=LINE ( 'NONE', #16063, #30878 ) ;
#15323=LINE ( 'NONE', #27814, #29117 ) ;
#15325=DIRECTION ( 'NONE',  ( 0.000000000000000000, 1.000000000000000000, 0.000000000000000000 ) ) ;
#15330=DIRECTION ( 'NONE',  ( -1.000000000000000000, 0.000000000000000000, 0.000000000000000000 ) ) ;
#15339=LINE ( 'NONE', #8837, #29568 ) ;
#15380=DIRECTION ( 'NONE',  ( 0.000000000000000000, -0.000000000000000000, 1.000000000000000000 ) ) ;
#15386=CARTESIAN_POINT ( 'NONE',  ( -177.4999999999999716, -72.50000000000001421, -9.999999999999973355 ) ) ;
#15396=ORIENTED_EDGE ( 'NONE', *, *, #3261, .T. ) ;
#15412=LINE ( 'NONE', #35184, #5085 ) ;
#15429=CARTESIAN_POINT ( 'NONE',  ( 0.000000000000000000, 0.000000000000000000, 790.0000000000000000 ) ) ;
#15469=LINE ( 'NONE', #10606, #3788 ) ;
#15483=VERTEX_POINT ( 'NONE', #46349 ) ;
#15488=VERTEX_POINT ( 'NONE', #43285 ) ;
#15490=ORIENTED_EDGE ( 'NONE', *, *, #21486, .T. ) ;
#15513=LINE ( 'NONE', #12175, #28652 ) ;
#15518=PLANE ( 'NONE',  #47519 ) ;
#15542=VECTOR ( 'NONE', #11031, 1000.000000000000000 ) ;
#15543=CARTESIAN_POINT ( 'NONE',  ( -37.90972275097263378, -14.83505920947805734, 901.8832493327278144 ) ) ;
#15556=FACE_OUTER_BOUND ( 'NONE', #23597, .T. ) ;
#15578=VECTOR ( 'NONE', #37124, 1000.000000000000114 ) ;
#15594=AXIS2_PLACEMENT_3D ( 'NONE', #4174, #35490, #50561 ) ;
#15645=ADVANCED_FACE ( 'NONE', ( #20700 ), #36376, .T. ) ;
#15656=DIRECTION ( 'NONE',  ( 0.000000000000000000, -1.000000000000000000, 0.000000000000000000 ) ) ;
#15661=ORIENTED_EDGE ( 'NONE', *, *, #26939, .F. ) ;
#15666=DIRECTION ( 'NONE',  ( 0.000000000000000000, -1.000000000000000000, 1.822804496942679766E-16 ) ) ;
#15698=LINE ( 'NONE', #3378, #36852 ) ;
#15702=CARTESIAN_POINT ( 'NONE',  ( -33.89193117067290473, 0.000000000000000000, 910.0000000000000000 ) ) ;
#15742=LINE ( 'NONE', #35268, #43025 ) ;
#15754=CARTESIAN_POINT ( 'NONE',  ( -376.8544389702902890, 164.9999999999999716, 219.8317560660027539 ) ) ;
#15775=EDGE_CURVE ( 'NONE', #16324, #48417, #5808, .T. ) ;
#15822=VECTOR ( 'NONE', #39768, 1000.000000000000000 ) ;
#15824=FACE_OUTER_BOUND ( 'NONE', #35065, .T. ) ;
#15836=FACE_BOUND ( 'NONE', #41434, .T. ) ;
#15837=CARTESIAN_POINT ( 'NONE',  ( -167.4999999999999432, 102.5000000000000142, 10.00000000000000000 ) ) ;
#15855=ORIENTED_EDGE ( 'NONE', *, *, #49656, .T. ) ;
#15867=DIRECTION ( 'NONE',  ( 0.000000000000000000, -0.000000000000000000, 1.000000000000000000 ) ) ;
#15871=LINE ( 'NONE', #35141, #29092 ) ;
#15872=LINE ( 'NONE', #19961, #24600 ) ;
#15881=DIRECTION ( 'NONE',  ( -1.000000000000000000, 0.000000000000000000, -0.000000000000000000 ) ) ;
#15888=EDGE_LOOP ( 'NONE', ( #10766, #32418, #5704, #13816 ) ) ;
#15900=AXIS2_PLACEMENT_3D ( 'NONE', #3270, #18917, #18665 ) ;
#15926=SHAPE_REPRESENTATION ( 'hopper', ( #45486 ), #11091 ) ;
#15947=EDGE_LOOP ( 'NONE', ( #28953, #14070, #34398, #18174 ) ) ;
#15961=AXIS2_PLACEMENT_3D ( 'NONE', #30094, #45951, #11087 ) ;
#15974=VECTOR ( 'NONE', #34598, 1000.000000000000000 ) ;
#15975=CARTESIAN_POINT ( 'NONE',  ( 224.9999999999999432, -175.0000000000000000, 32.29650858650035161 ) ) ;
#15989=VERTEX_POINT ( 'NONE', #18041 ) ;
#16003=LINE ( 'NONE', #9060, #26700 ) ;
#16015=CARTESIAN_POINT ( 'NONE',  ( 224.9999999999999716, -164.9999999999999716, 474.9999999999998863 ) ) ;
#16025=VECTOR ( 'NONE', #13529, 1000.000000000000000 ) ;
#16026=CARTESIAN_POINT ( 'NONE',  ( 177.5000000000000284, 112.5000000000000000, -10.00000000000000000 ) ) ;
#16033=VECTOR ( 'NONE', #36817, 1000.000000000000000 ) ;
#16059=ORIENTED_EDGE ( 'NONE', *, *, #17486, .F. ) ;
#16063=CARTESIAN_POINT ( 'NONE',  ( -239.0000000000000853, -165.6999999999999602, 254.8599999999999852 ) ) ;
#16113=VERTEX_POINT ( 'NONE', #48806 ) ;
#16122=CARTESIAN_POINT ( 'NONE',  ( 0.000000000000000000, -389.0218519071287346, 192.5658166940287970 ) ) ;
#16126=DIRECTION ( 'NONE',  ( 0.000000000000000000, -1.000000000000000000, 1.822804496942679766E-16 ) ) ;
#16156=ORIENTED_EDGE ( 'NONE', *, *, #42903, .F. ) ;
#16157=ADVANCED_FACE ( 'NONE', ( #3662 ), #30618, .T. ) ;
#16199=DIRECTION ( 'NONE',  ( 1.000000000000000000, 0.000000000000000000, 0.000000000000000000 ) ) ;
#16221=EDGE_CURVE ( 'NONE', #38683, #30983, #23945, .T. ) ;
#16222=EDGE_CURVE ( 'NONE', #24145, #33295, #30505, .T. ) ;
#16223=DIRECTION ( 'NONE',  ( 0.000000000000000000, 0.000000000000000000, -1.000000000000000000 ) ) ;
#16260=DIRECTION ( 'NONE',  ( -0.000000000000000000, 0.000000000000000000, 1.000000000000000000 ) ) ;
#16271=FACE_OUTER_BOUND ( 'NONE', #22079, .T. ) ;
#16285=EDGE_CURVE ( 'NONE', #18435, #4602, #35018, .T. ) ;
#16302=ORIENTED_EDGE ( 'NONE', *, *, #46857, .F. ) ;
#16303=FACE_OUTER_BOUND ( 'NONE', #17564, .T. ) ;
#16309=EDGE_CURVE ( 'NONE', #18068, #35388, #28046, .T. ) ;
#16323=VECTOR ( 'NONE', #43886, 1000.000000000000000 ) ;
#16324=VERTEX_POINT ( 'NONE', #21097 ) ;
#16357=DIRECTION ( 'NONE',  ( -1.000000000000000000, 0.000000000000000000, 0.000000000000000000 ) ) ;
#16360=AXIS2_PLACEMENT_3D ( 'NONE', #8589, #5234, #12423 ) ;
#16363=ORIENTED_EDGE ( 'NONE', *, *, #17913, .F. ) ;
#16373=CARTESIAN_POINT ( 'NONE',  ( 194.9999999999999432, 173.0000000000000000, 252.0000000000000000 ) ) ;
#16382=VECTOR ( 'NONE', #14622, 1000.000000000000000 ) ;
#16399=CARTESIAN_POINT ( 'NONE',  ( -214.9999999999999432, 173.0000000000000000, 112.0000000000000000 ) ) ;
#16405=EDGE_CURVE ( 'NONE', #42393, #15989, #32409, .T. ) ;
#16417=CARTESIAN_POINT ( 'NONE',  ( 224.9999999999999716, -164.9999999999999716, 62.29650858650038003 ) ) ;
#16449=VERTEX_POINT ( 'NONE', #22547 ) ;
#16452=FACE_OUTER_BOUND ( 'NONE', #18065, .T. ) ;
#16457=DIRECTION ( 'NONE',  ( -0.000000000000000000, -0.000000000000000000, 1.000000000000000000 ) ) ;
#16474=CIRCLE ( 'NONE', #8313, 40.00000000000000000 ) ;
#16477=EDGE_LOOP ( 'NONE', ( #40022, #42785, #10284, #42971, #24817, #41257 ) ) ;
#16490=VERTEX_POINT ( 'NONE', #46620 ) ;
#16521=DIRECTION ( 'NONE',  ( 1.000000000000000000, 0.000000000000000000, 0.000000000000000000 ) ) ;
#16526=CARTESIAN_POINT ( 'NONE',  ( 0.000000000000000000, 0.000000000000000000, 800.0000000000000000 ) ) ;
#16549=DIRECTION ( 'NONE',  ( -0.000000000000000000, -1.000000000000000000, 0.000000000000000000 ) ) ;
#16554=ORIENTED_EDGE ( 'NONE', *, *, #20260, .F. ) ;
#16555=ORIENTED_EDGE ( 'NONE', *, *, #15157, .T. ) ;
#16566=ORIENTED_EDGE ( 'NONE', *, *, #13918, .T. ) ;
#16573=ADVANCED_FACE ( 'NONE', ( #43310 ), #46874, .F. ) ;
#16577=EDGE_LOOP ( 'NONE', ( #2334, #30310, #13157, #10818 ) ) ;
#16604=VERTEX_POINT ( 'NONE', #4581 ) ;
#16638=VERTEX_POINT ( 'NONE', #43817 ) ;
#16643=ORIENTED_EDGE ( 'NONE', *, *, #22751, .T. ) ;
#16647=LINE ( 'NONE', #40763, #36964 ) ;
#16691=VECTOR ( 'NONE', #40087, 1000.000000000000114 ) ;
#16702=ADVANCED_FACE ( 'NONE', ( #5066 ), #9430, .T. ) ;
#16738=AXIS2_PLACEMENT_3D ( 'NONE', #18473, #10281, #30044 ) ;
#16741=EDGE_CURVE ( 'NONE', #18435, #23225, #25338, .T. ) ;
#16758=PLANE ( 'NONE',  #34039 ) ;
#16769=ORIENTED_EDGE ( 'NONE', *, *, #13758, .F. ) ;
#16795=DIRECTION ( 'NONE',  ( -0.000000000000000000, -0.000000000000000000, -1.000000000000000000 ) ) ;
#16816=DIRECTION ( 'NONE',  ( 1.000000000000000000, -0.000000000000000000, -0.000000000000000000 ) ) ;
#16817=DIRECTION ( 'NONE',  ( -0.000000000000000000, -1.000000000000000000, -0.000000000000000000 ) ) ;
#16851=VERTEX_POINT ( 'NONE', #22987 ) ;
#16862=DIRECTION ( 'NONE',  ( -0.000000000000000000, 1.604368532695312981E-16, 1.000000000000000000 ) ) ;
#16883=VECTOR ( 'NONE', #14359, 1000.000000000000000 ) ;
#16899=EDGE_CURVE ( 'NONE', #11165, #23532, #37612, .T. ) ;
#16902=UNCERTAINTY_MEASURE_WITH_UNIT (LENGTH_MEASURE( 1.000000000000000082E-05 ), #2311, 'distance_accuracy_value', 'NONE');
#16931=ORIENTED_EDGE ( 'NONE', *, *, #5778, .F. ) ;
#16939=LINE ( 'NONE', #9221, #209 ) ;
#16944=ORIENTED_EDGE ( 'NONE', *, *, #40314, .T. ) ;
#16959=CARTESIAN_POINT ( 'NONE',  ( 232.4999999999999716, -169.9999999999999716, 474.9999999999998863 ) ) ;
#16964=DIRECTION ( 'NONE',  ( 0.5038710255240862468, 0.000000000000000000, 0.8637789008984334549 ) ) ;
#16968=ORIENTED_EDGE ( 'NONE', *, *, #39308, .T. ) ;
#16971=LINE ( 'NONE', #25171, #42555 ) ;
#16984=EDGE_CURVE ( 'NONE', #42393, #639, #671, .T. ) ;
#16998=CARTESIAN_POINT ( 'NONE',  ( 0.000000000000000000, 33.89193117067290473, 910.0000000000000000 ) ) ;
#17041=VERTEX_POINT ( 'NONE', #19906 ) ;
#17070=DIRECTION ( 'NONE',  ( -0.9928768384869219865, 0.000000000000000000, -0.1191452206184307749 ) ) ;
#17096=CARTESIAN_POINT ( 'NONE',  ( 240.0000000000000000, -175.0000000000000000, 444.9999999999998295 ) ) ;
#17139=EDGE_CURVE ( 'NONE', #4161, #18435, #33495, .T. ) ;
#17141=PLANE ( 'NONE',  #679 ) ;
#17156=DIRECTION ( 'NONE',  ( 0.4055129968046615185, -0.4055129968046615185, -0.8192181753629524943 ) ) ;
#17183=VERTEX_POINT ( 'NONE', #32728 ) ;
#17213=ORIENTED_EDGE ( 'NONE', *, *, #18007, .F. ) ;
#17221=EDGE_LOOP ( 'NONE', ( #23851, #29486, #49988, #36437, #44988 ) ) ;
#17222=DIRECTION ( 'NONE',  ( 0.000000000000000000, -1.000000000000000000, 2.406552799042969348E-16 ) ) ;
#17246=DIRECTION ( 'NONE',  ( 0.000000000000000000, -1.000000000000000000, 1.604368532695312981E-16 ) ) ;
#17259=LINE ( 'NONE', #13151, #43902 ) ;
#17277=DIRECTION ( 'NONE',  ( 0.000000000000000000, -0.000000000000000000, 1.000000000000000000 ) ) ;
#17287=EDGE_LOOP ( 'NONE', ( #21700, #46426, #16363, #36527 ) ) ;
#17298=ORIENTED_EDGE ( 'NONE', *, *, #40091, .T. ) ;
#17308=DIRECTION ( 'NONE',  ( -0.1191452206184307749, 0.000000000000000000, 0.9928768384869220975 ) ) ;
#17316=DIRECTION ( 'NONE',  ( -0.000000000000000000, -0.000000000000000000, -1.000000000000000000 ) ) ;
#17341=ORIENTED_EDGE ( 'NONE', *, *, #1387, .T. ) ;
#17351=ORIENTED_EDGE ( 'NONE', *, *, #35942, .T. ) ;
#17360=VERTEX_POINT ( 'NONE', #30917 ) ;
#17367=DIRECTION ( 'NONE',  ( -0.9928768384869220975, 0.000000000000000000, -0.1191452206184309970 ) ) ;
#17376=ADVANCED_FACE ( 'NONE', ( #11653, #8320 ), #7554, .T. ) ;
#17403=VECTOR ( 'NONE', #43862, 1000.000000000000000 ) ;
#17424=CARTESIAN_POINT ( 'NONE',  ( -167.4999999999999432, -62.49999999999998579, -10.00000000000000000 ) ) ;
#17452=EDGE_LOOP ( 'NONE', ( #16302, #19775, #39038, #9226 ) ) ;
#17459=EDGE_CURVE ( 'NONE', #44566, #36764, #3947, .T. ) ;
#17481=PLANE ( 'NONE',  #38543 ) ;
#17486=EDGE_CURVE ( 'NONE', #49286, #9722, #33189, .T. ) ;
#17503=ORIENTED_EDGE ( 'NONE', *, *, #8254, .T. ) ;
#17504=AXIS2_PLACEMENT_3D ( 'NONE', #33250, #44497, #25037 ) ;
#17513=CARTESIAN_POINT ( 'NONE',  ( -50.00000000000000000, 50.00000000000000000, 900.0000000000000000 ) ) ;
#17518=DIRECTION ( 'NONE',  ( -1.000000000000000000, -0.000000000000000000, -0.000000000000000000 ) ) ;
#17551=ADVANCED_FACE ( 'NONE', ( #28818 ), #44439, .T. ) ;
#17564=EDGE_LOOP ( 'NONE', ( #44991, #36940, #50339, #5321 ) ) ;
#17571=CARTESIAN_POINT ( 'NONE',  ( 240.0000000000000000, -175.0000000000000000, 32.29650858650035161 ) ) ;
#17585=VECTOR ( 'NONE', #32654, 1000.000000000000000 ) ;
#17618=CARTESIAN_POINT ( 'NONE',  ( 40.00000000000000000, -7.564790863224926554, 897.6604670114604687 ) ) ;
#17630=CARTESIAN_POINT ( 'NONE',  ( -50.00000000000000000, -50.00000000000000000, 900.0000000000000000 ) ) ;
#17631=AXIS2_PLACEMENT_3D ( 'NONE', #31250, #200, #34852 ) ;
#17659=LINE ( 'NONE', #49421, #24204 ) ;
#17673=EDGE_CURVE ( 'NONE', #25022, #19653, #11076, .T. ) ;
#17677=VERTEX_POINT ( 'NONE', #38305 ) ;
#17683=PLANE ( 'NONE',  #6253 ) ;
#17706=EDGE_CURVE ( 'NONE', #29488, #11677, #18762, .T. ) ;
#17835=CARTESIAN_POINT ( 'NONE',  ( -215.0000000000000568, -172.9999999999999716, 252.0000000000000000 ) ) ;
#17837=ADVANCED_FACE ( 'NONE', ( #1559, #16452 ), #40806, .F. ) ;
#17842=ORIENTED_EDGE ( 'NONE', *, *, #28204, .T. ) ;
#17847=DIRECTION ( 'NONE',  ( -0.9908916497796512735, 0.000000000000000000, -0.1346615698592613652 ) ) ;
#17880=CYLINDRICAL_SURFACE ( 'NONE', #28519, 3.500000000000003109 ) ;
#17884=ADVANCED_FACE ( 'NONE', ( #29001 ), #44621, .F. ) ;
#17902=AXIS2_PLACEMENT_3D ( 'NONE', #36869, #48081, #32239 ) ;
#17907=PLANE ( 'NONE',  #1573 ) ;
#17913=EDGE_CURVE ( 'NONE', #42445, #27283, #24909, .T. ) ;
#17914=CARTESIAN_POINT ( 'NONE',  ( 194.9999999999999432, -172.9999999999999716, 252.0000000000000568 ) ) ;
#17937=LINE ( 'NONE', #45874, #16883 ) ;
#17945=AXIS2_PLACEMENT_3D ( 'NONE', #49409, #6352, #18394 ) ;
#17955=ORIENTED_EDGE ( 'NONE', *, *, #13987, .T. ) ;
#17959=FACE_OUTER_BOUND ( 'NONE', #18317, .T. ) ;
#18007=EDGE_CURVE ( 'NONE', #639, #16638, #17937, .T. ) ;
#18008=EDGE_CURVE ( 'NONE', #9652, #50112, #45632, .T. ) ;
#18028=VECTOR ( 'NONE', #13081, 1000.000000000000000 ) ;
#18041=CARTESIAN_POINT ( 'NONE',  ( -177.4999999999999716, -112.5000000000000000, -9.999999999999973355 ) ) ;
#18045=ORIENTED_EDGE ( 'NONE', *, *, #49269, .T. ) ;
#18065=EDGE_LOOP ( 'NONE', ( #3418, #46354, #28542, #24928 ) ) ;
#18067=CIRCLE ( 'NONE', #36973, 3.500000000000003109 ) ;
#18068=VERTEX_POINT ( 'NONE', #19730 ) ;
#18087=DIRECTION ( 'NONE',  ( -1.000000000000000000, -0.000000000000000000, -0.000000000000000000 ) ) ;
#18107=LINE ( 'NONE', #3201, #49466 ) ;
#18109=ORIENTED_EDGE ( 'NONE', *, *, #24146, .F. ) ;
#18135=LINE ( 'NONE', #15055, #24003 ) ;
#18137=DIRECTION ( 'NONE',  ( -0.000000000000000000, -0.000000000000000000, 1.000000000000000000 ) ) ;
#18144=CARTESIAN_POINT ( 'NONE',  ( 224.9999999999999716, -164.9999999999999716, 474.9999999999998863 ) ) ;
#18165=CARTESIAN_POINT ( 'NONE',  ( 389.0218519071287346, 0.000000000000000000, 192.5658166940287970 ) ) ;
#18174=ORIENTED_EDGE ( 'NONE', *, *, #12716, .F. ) ;
#18181=EDGE_CURVE ( 'NONE', #4421, #28864, #7943, .T. ) ;
#18248=ORIENTED_EDGE ( 'NONE', *, *, #539, .T. ) ;
#18252=PLANE ( 'NONE',  #13838 ) ;
#18273=CARTESIAN_POINT ( 'NONE',  ( -225.0000000000000568, -175.0000000000000000, 0.000000000000000000 ) ) ;
#18276=ORIENTED_EDGE ( 'NONE', *, *, #3989, .T. ) ;
#18277=CARTESIAN_POINT ( 'NONE',  ( -239.0000000000000853, -153.6999999999999602, 250.3600000000000136 ) ) ;
#18292=VERTEX_POINT ( 'NONE', #44764 ) ;
#18298=EDGE_CURVE ( 'NONE', #20787, #13604, #36870, .T. ) ;
#18317=EDGE_LOOP ( 'NONE', ( #36156, #25998, #398 ) ) ;
#18324=EDGE_CURVE ( 'NONE', #18292, #50400, #7297, .T. ) ;
#18332=CARTESIAN_POINT ( 'NONE',  ( 0.000000000000000000, 0.000000000000000000, 800.0000000000000000 ) ) ;
#18335=LINE ( 'NONE', #49842, #36360 ) ;
#18340=ORIENTED_EDGE ( 'NONE', *, *, #16899, .F. ) ;
#18357=ORIENTED_EDGE ( 'NONE', *, *, #3989, .F. ) ;
#18377=DIRECTION ( 'NONE',  ( -1.000000000000000000, 0.000000000000000000, 0.000000000000000000 ) ) ;
#18390=EDGE_CURVE ( 'NONE', #36453, #33652, #5290, .T. ) ;
#18394=DIRECTION ( 'NONE',  ( 1.000000000000000000, 0.000000000000000000, 0.000000000000000000 ) ) ;
#18397=LINE ( 'NONE', #18144, #5843 ) ;
#18401=CARTESIAN_POINT ( 'NONE',  ( -177.4999999999999716, 57.49999999999996447, -9.999999999999973355 ) ) ;
#18417=DIRECTION ( 'NONE',  ( 0.000000000000000000, 0.000000000000000000, -1.000000000000000000 ) ) ;
#18424=LINE ( 'NONE', #30489, #15974 ) ;
#18435=VERTEX_POINT ( 'NONE', #42944 ) ;
#18452=EDGE_CURVE ( 'NONE', #48180, #35326, #4723, .T. ) ;
#18463=ADVANCED_FACE ( 'NONE', ( #4466 ), #50608, .F. ) ;
#18473=CARTESIAN_POINT ( 'NONE',  ( 0.000000000000000000, 0.000000000000000000, 900.0000000000000000 ) ) ;
#18493=CARTESIAN_POINT ( 'NONE',  ( -225.0000000000000284, 175.0000000000000000, 500.0000000000000000 ) ) ;
#18506=ORIENTED_EDGE ( 'NONE', *, *, #39267, .T. ) ;
#18507=VECTOR ( 'NONE', #19945, 1000.000000000000000 ) ;
#18512=CARTESIAN_POINT ( 'NONE',  ( 194.9999999999999432, -173.0000000000000000, 112.0000000000000284 ) ) ;
#18529=PLANE ( 'NONE',  #22960 ) ;
#18556=DIRECTION ( 'NONE',  ( -1.000000000000000000, -0.000000000000000000, -0.000000000000000000 ) ) ;
#18566=FACE_OUTER_BOUND ( 'NONE', #40691, .T. ) ;
#18616=CARTESIAN_POINT ( 'NONE',  ( 37.90972275097264088, 14.83505920947803070, 901.8832493327278144 ) ) ;
#18617=CARTESIAN_POINT ( 'NONE',  ( -50.00000000000000000, 50.00000000000000000, 800.0000000000000000 ) ) ;
#18629=DIRECTION ( 'NONE',  ( 1.000000000000000000, 0.000000000000000000, 0.000000000000000000 ) ) ;
#18640=ADVANCED_FACE ( 'NONE', ( #18771 ), #14433, .F. ) ;
#18646=EDGE_CURVE ( 'NONE', #44943, #49618, #13489, .T. ) ;
#18665=DIRECTION ( 'NONE',  ( 0.000000000000000000, 0.000000000000000000, 1.000000000000000000 ) ) ;
#18722=LINE ( 'NONE', #42339, #22107 ) ;
#18726=ORIENTED_EDGE ( 'NONE', *, *, #5008, .F. ) ;
#18733=DIRECTION ( 'NONE',  ( -0.4740998230350175202, 0.3386427307392980146, -0.8127425537743157014 ) ) ;
#18746=DIRECTION ( 'NONE',  ( -1.000000000000000000, 0.000000000000000000, 0.000000000000000000 ) ) ;
#18762=LINE ( 'NONE', #6465, #29149 ) ;
#18771=FACE_OUTER_BOUND ( 'NONE', #27969, .T. ) ;
#18785=DIRECTION ( 'NONE',  ( 1.000000000000000000, -0.000000000000000000, -0.000000000000000000 ) ) ;
#18789=EDGE_LOOP ( 'NONE', ( #39896, #44286, #29870, #31967, #28496, #24131, #31095, #50347 ) ) ;
#18794=ORIENTED_EDGE ( 'NONE', *, *, #10461, .F. ) ;
#18802=CARTESIAN_POINT ( 'NONE',  ( -568.6915979970481203, -62.49999999999998579, -173.6700166912652890 ) ) ;
#18824=DIRECTION ( 'NONE',  ( 0.9908916497796512735, -0.000000000000000000, 0.1346615698592613375 ) ) ;
#18840=DIRECTION ( 'NONE',  ( 0.4740998230350171871, 0.3386427307392981256, -0.8127425537743158124 ) ) ;
#18843=VECTOR ( 'NONE', #4306, 1000.000000000000000 ) ;
#18876=DIRECTION ( 'NONE',  ( -0.000000000000000000, 0.000000000000000000, 1.000000000000000000 ) ) ;
#18917=DIRECTION ( 'NONE',  ( 0.000000000000000000, 1.000000000000000000, -0.000000000000000000 ) ) ;
#18924=CARTESIAN_POINT ( 'NONE',  ( -225.0000000000000568, -165.6999999999999602, 250.3600000000000136 ) ) ;
#18930=VERTEX_POINT ( 'NONE', #9012 ) ;
#18931=ORIENTED_EDGE ( 'NONE', *, *, #41962, .F. ) ;
#18938=EDGE_CURVE ( 'NONE', #35427, #30532, #9504, .T. ) ;
#18939=CARTESIAN_POINT ( 'NONE',  ( -214.9999999999999432, -173.0000000000000000, 112.0000000000000284 ) ) ;
#18946=DIRECTION ( 'NONE',  ( 0.000000000000000000, 8.021842663476564905E-17, 1.000000000000000000 ) ) ;
#18948=VERTEX_POINT ( 'NONE', #43894 ) ;
#18954=PLANE ( 'NONE',  #36330 ) ;
#19029=FACE_OUTER_BOUND ( 'NONE', #22291, .T. ) ;
#19047=CARTESIAN_POINT ( 'NONE',  ( -44.25629667545849344, -43.33333333333336412, 790.0000000000000000 ) ) ;
#19082=VERTEX_POINT ( 'NONE', #10273 ) ;
#19148=AXIS2_PLACEMENT_3D ( 'NONE', #34630, #7681, #15380 ) ;
#19159=LINE ( 'NONE', #30994, #34490 ) ;
#19166=ORIENTED_EDGE ( 'NONE', *, *, #24632, .F. ) ;
#19176=CARTESIAN_POINT ( 'NONE',  ( -177.4999999999999716, -72.50000000000001421, -130.5992382549688671 ) ) ;
#19192=LINE ( 'NONE', #43814, #6736 ) ;
#19253=VECTOR ( 'NONE', #25465, 1000.000000000000000 ) ;
#19268=ORIENTED_EDGE ( 'NONE', *, *, #25570, .T. ) ;
#19275=VECTOR ( 'NONE', #11723, 1000.000000000000000 ) ;
#19344=CARTESIAN_POINT ( 'NONE',  ( -194.9999999999999432, -173.0000000000000000, 372.0000000000000568 ) ) ;
#19363=CARTESIAN_POINT ( 'NONE',  ( -376.8544389702902890, 0.000000000000000000, 219.8317560660027539 ) ) ;
#19382=ORIENTED_EDGE ( 'NONE', *, *, #8632, .F. ) ;
#19385=EDGE_LOOP ( 'NONE', ( #11606, #4729, #45972, #4203 ) ) ;
#19425=CARTESIAN_POINT ( 'NONE',  ( -177.4999999999999716, 57.49999999999996447, -9.999999999999973355 ) ) ;
#19429=PLANE ( 'NONE',  #24155 ) ;
#19451=DIRECTION ( 'NONE',  ( 0.9908916497796512735, 0.000000000000000000, 0.1346615698592613375 ) ) ;
#19452=CARTESIAN_POINT ( 'NONE',  ( -225.0000000000000568, 175.0000000000000000, 0.000000000000000000 ) ) ;
#19463=CARTESIAN_POINT ( 'NONE',  ( 194.9999999999999432, -173.0000000000000000, 372.0000000000000568 ) ) ;
#19468=CARTESIAN_POINT ( 'NONE',  ( -167.4999999999999432, 67.47808924524055385, -120.5992382549688955 ) ) ;
#19493=LINE ( 'NONE', #35181, #9341 ) ;
#19515=ORIENTED_EDGE ( 'NONE', *, *, #3691, .T. ) ;
#19522=DIRECTION ( 'NONE',  ( 1.000000000000000000, 0.000000000000000000, 0.000000000000000000 ) ) ;
#19534=ORIENTED_EDGE ( 'NONE', *, *, #2640, .T. ) ;
#19536=DIRECTION ( 'NONE',  ( 0.000000000000000000, 0.000000000000000000, 1.000000000000000000 ) ) ;
#19542=DIRECTION ( 'NONE',  ( 0.000000000000000000, -0.000000000000000000, 1.000000000000000000 ) ) ;
#19562=FACE_OUTER_BOUND ( 'NONE', #16577, .T. ) ;
#19576=EDGE_LOOP ( 'NONE', ( #30814, #29218, #21370, #42928 ) ) ;
#19598=CYLINDRICAL_SURFACE ( 'NONE', #43589, 40.00000000000000000 ) ;
#19605=EDGE_CURVE ( 'NONE', #4495, #44090, #35098, .T. ) ;
#19634=ORIENTED_EDGE ( 'NONE', *, *, #13464, .T. ) ;
#19653=VERTEX_POINT ( 'NONE', #36623 ) ;
#19655=CARTESIAN_POINT ( 'NONE',  ( -225.0000000000000568, 164.9999999999999716, 231.9999999999999716 ) ) ;
#19673=AXIS2_PLACEMENT_3D ( 'NONE', #30672, #46268, #45769 ) ;
#19703=LINE ( 'NONE', #18924, #39018 ) ;
#19707=CARTESIAN_POINT ( 'NONE',  ( 167.5000000000000000, -102.5000000000000142, -8.575805527524005711 ) ) ;
#19730=CARTESIAN_POINT ( 'NONE',  ( 214.9999999999999432, 164.9999999999999716, 352.0000000000000000 ) ) ;
#19744=ORIENTED_EDGE ( 'NONE', *, *, #13283, .T. ) ;
#19749=ORIENTED_EDGE ( 'NONE', *, *, #22527, .T. ) ;
#19766=CARTESIAN_POINT ( 'NONE',  ( 224.9999999999999716, -164.9999999999999716, 32.29650858650035161 ) ) ;
#19775=ORIENTED_EDGE ( 'NONE', *, *, #36185, .F. ) ;
#19842=EDGE_CURVE ( 'NONE', #30983, #30113, #24329, .T. ) ;
#19868=EDGE_CURVE ( 'NONE', #36027, #4421, #39725, .T. ) ;
#19906=CARTESIAN_POINT ( 'NONE',  ( -215.0000000000000568, -173.0000000000000000, 132.0000000000001137 ) ) ;
#19912=CARTESIAN_POINT ( 'NONE',  ( 214.9999999999999432, 0.000000000000000000, 10.00000000000000000 ) ) ;
#19936=DIRECTION ( 'NONE',  ( 0.000000000000000000, 0.000000000000000000, -1.000000000000000000 ) ) ;
#19944=FACE_OUTER_BOUND ( 'NONE', #33979, .T. ) ;
#19945=DIRECTION ( 'NONE',  ( 0.000000000000000000, 1.000000000000000000, 0.000000000000000000 ) ) ;
#19951=ORIENTED_EDGE ( 'NONE', *, *, #32744, .F. ) ;
#19954=EDGE_LOOP ( 'NONE', ( #50428, #29630, #26178, #8913 ) ) ;
#19957=FACE_OUTER_BOUND ( 'NONE', #6775, .T. ) ;
#19961=CARTESIAN_POINT ( 'NONE',  ( 214.9999999999999432, 164.9999999999999716, 500.0000000000000000 ) ) ;
#19985=LINE ( 'NONE', #47645, #41689 ) ;
#19997=CARTESIAN_POINT ( 'NONE',  ( -239.0000000000000853, -165.6999999999999602, 250.3600000000000136 ) ) ;
#19999=ORIENTED_EDGE ( 'NONE', *, *, #14208, .F. ) ;
#20004=DIRECTION ( 'NONE',  ( 0.000000000000000000, 0.000000000000000000, 1.000000000000000000 ) ) ;
#20007=DIRECTION ( 'NONE',  ( 0.000000000000000000, 0.000000000000000000, 1.000000000000000000 ) ) ;
#20018=ORIENTED_EDGE ( 'NONE', *, *, #28962, .F. ) ;
#20032=DIRECTION ( 'NONE',  ( -0.000000000000000000, -0.000000000000000000, -1.000000000000000000 ) ) ;
#20034=( BOUNDED_CURVE ( )  B_SPLINE_CURVE ( 3, ( #3737, #50639, #15543, #46793 ),
 .UNSPECIFIED., .F., .F. ) 
 B_SPLINE_CURVE_WITH_KNOTS ( ( 4, 4 ),
 ( 0.000000000000000000, 0.5599187270832629570 ),
 .UNSPECIFIED. ) 
 CURVE ( )  GEOMETRIC_REPRESENTATION_ITEM ( )  RATIONAL_B_SPLINE_CURVE ( ( 1.000000000000000000, 0.9740444450880465510, 0.9740444450880465510, 1.000000000000000000 ) ) 
 REPRESENTATION_ITEM ( '' )  );
#20043=CARTESIAN_POINT ( 'NONE',  ( -239.0000000000000853, -165.6999999999999602, 250.3600000000000136 ) ) ;
#20049=DIRECTION ( 'NONE',  ( 0.000000000000000000, 0.000000000000000000, 1.000000000000000000 ) ) ;
#20067=DIRECTION ( 'NONE',  ( 0.000000000000000000, -0.9602398687205827565, -0.2791762785758810650 ) ) ;
#20082=CARTESIAN_POINT ( 'NONE',  ( -50.00000000000000000, 50.00000000000000000, 800.0000000000000000 ) ) ;
#20091=CARTESIAN_POINT ( 'NONE',  ( -21.24469349090191983, -33.89193117067290473, 910.0000000000000000 ) ) ;
#20092=LINE ( 'NONE', #8559, #21790 ) ;
#20112=DIRECTION ( 'NONE',  ( -1.000000000000000000, 0.000000000000000000, -0.000000000000000000 ) ) ;
#20122=CARTESIAN_POINT ( 'NONE',  ( -50.00000000000000000, -50.00000000000000000, 900.0000000000000000 ) ) ;
#20129=DIRECTION ( 'NONE',  ( 0.000000000000000000, -1.000000000000000000, 0.000000000000000000 ) ) ;
#20169=EDGE_CURVE ( 'NONE', #12891, #38992, #28600, .T. ) ;
#20180=VECTOR ( 'NONE', #7525, 1000.000000000000000 ) ;
#20189=ORIENTED_EDGE ( 'NONE', *, *, #11528, .T. ) ;
#20198=ADVANCED_FACE ( 'NONE', ( #16303 ), #4750, .T. ) ;
#20205=ADVANCED_FACE ( 'NONE', ( #48565 ), #49065, .T. ) ;
#20212=EDGE_LOOP ( 'NONE', ( #23510, #7646, #32441, #29445 ) ) ;
#20260=EDGE_CURVE ( 'NONE', #32080, #8986, #32713, .T. ) ;
#20272=EDGE_CURVE ( 'NONE', #47971, #29800, #13201, .T. ) ;
#20324=( BOUNDED_CURVE ( )  B_SPLINE_CURVE ( 3, ( #38923, #34555, #3749, #35084 ),
 .UNSPECIFIED., .F., .F. ) 
 B_SPLINE_CURVE_WITH_KNOTS ( ( 4, 4 ),
 ( 5.723266580096323608, 6.843104034262848856 ),
 .UNSPECIFIED. ) 
 CURVE ( )  GEOMETRIC_REPRESENTATION_ITEM ( )  RATIONAL_B_SPLINE_CURVE ( ( 1.000000000000000000, 0.8981988528445483677, 0.8981988528445483677, 1.000000000000000000 ) ) 
 REPRESENTATION_ITEM ( '' )  );
#20358=VERTEX_POINT ( 'NONE', #18802 ) ;
#20371=VECTOR ( 'NONE', #9381, 1000.000000000000000 ) ;
#20378=ORIENTED_EDGE ( 'NONE', *, *, #26518, .T. ) ;
#20384=CARTESIAN_POINT ( 'NONE',  ( -225.0000000000000568, 0.000000000000000000, 500.0000000000000000 ) ) ;
#20392=CARTESIAN_POINT ( 'NONE',  ( 194.9999999999999432, 0.000000000000000000, 0.000000000000000000 ) ) ;
#20417=EDGE_CURVE ( 'NONE', #10351, #16113, #22667, .T. ) ;
#20426=ORIENTED_EDGE ( 'NONE', *, *, #26542, .F. ) ;
#20445=CARTESIAN_POINT ( 'NONE',  ( -50.00000000000000000, 50.00000000000000000, 900.0000000000000000 ) ) ;
#20463=LINE ( 'NONE', #44543, #46260 ) ;
#20508=ORIENTED_EDGE ( 'NONE', *, *, #27707, .T. ) ;
#20524=LINE ( 'NONE', #4632, #26972 ) ;
#20543=EDGE_LOOP ( 'NONE', ( #28325, #36788, #26196, #23216, #2283 ) ) ;
#20546=CARTESIAN_POINT ( 'NONE',  ( -44.25629667545849344, 0.000000000000000000, 790.0000000000000000 ) ) ;
#20555=EDGE_CURVE ( 'NONE', #49286, #26731, #35506, .T. ) ;
#20583=DIRECTION ( 'NONE',  ( 0.1191452206184309970, 0.000000000000000000, -0.9928768384869220975 ) ) ;
#20598=PLANE ( 'NONE',  #50208 ) ;
#20601=AXIS2_PLACEMENT_3D ( 'NONE', #41390, #19542, #39323 ) ;
#20609=EDGE_CURVE ( 'NONE', #5026, #14784, #48250, .T. ) ;
#20611=CARTESIAN_POINT ( 'NONE',  ( 224.9999999999999716, -164.9999999999999716, 32.29650858650035161 ) ) ;
#20633=VECTOR ( 'NONE', #20049, 1000.000000000000000 ) ;
#20634=PLANE ( 'NONE',  #31236 ) ;
#20648=VERTEX_POINT ( 'NONE', #1608 ) ;
#20663=LINE ( 'NONE', #49577, #9227 ) ;
#20665=CARTESIAN_POINT ( 'NONE',  ( -177.4999999999999716, -72.50000000000001421, -9.999999999999973355 ) ) ;
#20700=FACE_OUTER_BOUND ( 'NONE', #15947, .T. ) ;
#20703=LINE ( 'NONE', #43791, #9022 ) ;
#20787=VERTEX_POINT ( 'NONE', #37778 ) ;
#20876=ORIENTED_EDGE ( 'NONE', *, *, #19868, .F. ) ;
#20892=VECTOR ( 'NONE', #35367, 1000.000000000000000 ) ;
#20913=DIRECTION ( 'NONE',  ( -0.000000000000000000, -1.000000000000000000, -0.000000000000000000 ) ) ;
#20996=LINE ( 'NONE', #12785, #29823 ) ;
#21018=ORIENTED_EDGE ( 'NONE', *, *, #12100, .F. ) ;
#21044=ORIENTED_EDGE ( 'NONE', *, *, #2486, .F. ) ;
#21061=ORIENTED_EDGE ( 'NONE', *, *, #29955, .F. ) ;
#21070=ORIENTED_EDGE ( 'NONE', *, *, #43141, .F. ) ;
#21086=EDGE_CURVE ( 'NONE', #31054, #13689, #30029, .T. ) ;
#21097=CARTESIAN_POINT ( 'NONE',  ( -167.4999999999999432, -62.49999999999998579, -18.87174264961130987 ) ) ;
#21101=DIRECTION ( 'NONE',  ( 0.8637789008984335659, -0.000000000000000000, 0.5038710255240859137 ) ) ;
#21120=EDGE_CURVE ( 'NONE', #16449, #18930, #23763, .T. ) ;
#21136=LINE ( 'NONE', #49296, #16033 ) ;
#21138=ORIENTED_EDGE ( 'NONE', *, *, #45707, .F. ) ;
#21145=ORIENTED_EDGE ( 'NONE', *, *, #2475, .F. ) ;
#21153=EDGE_CURVE ( 'NONE', #34586, #30983, #15311, .T. ) ;
#21176=LINE ( 'NONE', #39941, #20371 ) ;
#21196=FACE_OUTER_BOUND ( 'NONE', #38858, .T. ) ;
#21204=DIRECTION ( 'NONE',  ( 0.000000000000000000, 0.000000000000000000, 1.000000000000000000 ) ) ;
#21216=ORIENTED_EDGE ( 'NONE', *, *, #22678, .T. ) ;
#21268=ORIENTED_EDGE ( 'NONE', *, *, #8254, .F. ) ;
#21284=AXIS2_PLACEMENT_3D ( 'NONE', #9970, #48917, #18417 ) ;
#21289=CARTESIAN_POINT ( 'NONE',  ( 214.9999999999999432, 164.9999999999999716, 252.0000000000000000 ) ) ;
#21292=DIRECTION ( 'NONE',  ( -1.000000000000000000, 0.000000000000000000, 0.000000000000000000 ) ) ;
#21294=VECTOR ( 'NONE', #10306, 1000.000000000000000 ) ;
#21300=DIRECTION ( 'NONE',  ( 0.000000000000000000, -0.000000000000000000, -1.000000000000000000 ) ) ;
#21336=DIRECTION ( 'NONE',  ( -0.000000000000000000, 0.8962124318248270161, 0.4436251537532894806 ) ) ;
#21359=CARTESIAN_POINT ( 'NONE',  ( 0.000000000000000000, 0.000000000000000000, 900.0000000000000000 ) ) ;
#21370=ORIENTED_EDGE ( 'NONE', *, *, #26542, .T. ) ;
#21432=CARTESIAN_POINT ( 'NONE',  ( -167.4999999999999432, -102.5000000000000142, -10.00000000000000000 ) ) ;
#21442=CARTESIAN_POINT ( 'NONE',  ( -215.0000000000000568, 164.9999999999999716, 500.0000000000000000 ) ) ;
#21454=EDGE_CURVE ( 'NONE', #3211, #32080, #20092, .T. ) ;
#21462=AXIS2_PLACEMENT_3D ( 'NONE', #39130, #46757, #3953 ) ;
#21476=DIRECTION ( 'NONE',  ( -1.000000000000000000, 0.000000000000000000, 0.000000000000000000 ) ) ;
#21482=DIRECTION ( 'NONE',  ( 0.000000000000000000, 0.000000000000000000, -1.000000000000000000 ) ) ;
#21486=EDGE_CURVE ( 'NONE', #4602, #10114, #16003, .T. ) ;
#21510=ORIENTED_EDGE ( 'NONE', *, *, #24041, .F. ) ;
#21532=EDGE_CURVE ( 'NONE', #22974, #12746, #48508, .T. ) ;
#21537=EDGE_CURVE ( 'NONE', #16851, #18292, #17259, .T. ) ;
#21571=CARTESIAN_POINT ( 'NONE',  ( -215.0000000000000568, 164.9999999999999716, 352.0000000000000000 ) ) ;
#21580=ORIENTED_EDGE ( 'NONE', *, *, #39450, .T. ) ;
#21608=ORIENTED_EDGE ( 'NONE', *, *, #16309, .F. ) ;
#21611=ORIENTED_EDGE ( 'NONE', *, *, #5152, .T. ) ;
#21627=CARTESIAN_POINT ( 'NONE',  ( 21.24469349090191983, -33.89193117067290473, 910.0000000000000000 ) ) ;
#21641=VECTOR ( 'NONE', #44980, 1000.000000000000000 ) ;
#21653=LINE ( 'NONE', #5746, #27250 ) ;
#21664=CARTESIAN_POINT ( 'NONE',  ( -194.9999999999999432, -173.0000000000000000, 112.0000000000000284 ) ) ;
#21684=CARTESIAN_POINT ( 'NONE',  ( 228.9999999999999716, -169.9999999999999716, 444.9999999999998295 ) ) ;
#21700=ORIENTED_EDGE ( 'NONE', *, *, #14056, .F. ) ;
#21715=CARTESIAN_POINT ( 'NONE',  ( -582.5000000000000000, 57.49999999999996447, -58.60000000000003695 ) ) ;
#21734=DIRECTION ( 'NONE',  ( 0.000000000000000000, -1.604368532695312981E-16, -1.000000000000000000 ) ) ;
#21738=AXIS2_PLACEMENT_3D ( 'NONE', #16015, #16260, #31925 ) ;
#21751=EDGE_CURVE ( 'NONE', #9008, #16851, #43881, .T. ) ;
#21771=DIRECTION ( 'NONE',  ( -1.000000000000000000, 0.000000000000000000, -0.000000000000000000 ) ) ;
#21773=VECTOR ( 'NONE', #31965, 1000.000000000000000 ) ;
#21790=VECTOR ( 'NONE', #40115, 1000.000000000000000 ) ;
#21793=CARTESIAN_POINT ( 'NONE',  ( -167.4999999999999716, -102.8976013127941656, -7.208237214241163926 ) ) ;
#21810=CARTESIAN_POINT ( 'NONE',  ( -215.0000000000000568, 164.9999999999999716, 500.0000000000000000 ) ) ;
#21827=VERTEX_POINT ( 'NONE', #48447 ) ;
#21848=CARTESIAN_POINT ( 'NONE',  ( 177.5000000000000284, 112.5000000000000000, -10.00000000000000000 ) ) ;
#21908=ORIENTED_EDGE ( 'NONE', *, *, #5545, .T. ) ;
#21920=DIRECTION ( 'NONE',  ( 0.9928768384869219865, 0.000000000000000000, 0.1191452206184307611 ) ) ;
#21923=ORIENTED_EDGE ( 'NONE', *, *, #5614, .T. ) ;
#21924=ORIENTED_EDGE ( 'NONE', *, *, #17706, .F. ) ;
#21939=DIRECTION ( 'NONE',  ( 0.000000000000000000, 0.9545212652235329776, -0.2981428420003837121 ) ) ;
#21950=VERTEX_POINT ( 'NONE', #34622 ) ;
#21984=DIRECTION ( 'NONE',  ( 0.000000000000000000, -0.000000000000000000, 1.000000000000000000 ) ) ;
#22016=CARTESIAN_POINT ( 'NONE',  ( 0.000000000000000000, 0.000000000000000000, 1000.000000000000000 ) ) ;
#22051=CIRCLE ( 'NONE', #49861, 3.500000000000003109 ) ;
#22079=EDGE_LOOP ( 'NONE', ( #41674, #38648, #6216, #11793 ) ) ;
#22107=VECTOR ( 'NONE', #34664, 1000.000000000000000 ) ;
#22126=LINE ( 'NONE', #10825, #42811 ) ;
#22141=VECTOR ( 'NONE', #19451, 1000.000000000000114 ) ;
#22142=FACE_OUTER_BOUND ( 'NONE', #403, .T. ) ;
#22153=ADVANCED_FACE ( 'NONE', ( #44310 ), #1990, .T. ) ;
#22156=DIRECTION ( 'NONE',  ( -0.000000000000000000, -0.000000000000000000, -1.000000000000000000 ) ) ;
#22184=CARTESIAN_POINT ( 'NONE',  ( 0.000000000000000000, 0.000000000000000000, 910.0000000000000000 ) ) ;
#22193=DIRECTION ( 'NONE',  ( -0.000000000000000000, -0.000000000000000000, 1.000000000000000000 ) ) ;
#22229=EDGE_CURVE ( 'NONE', #39414, #47971, #10193, .T. ) ;
#22246=ORIENTED_EDGE ( 'NONE', *, *, #45597, .T. ) ;
#22277=LINE ( 'NONE', #26117, #14760 ) ;
#22282=FACE_OUTER_BOUND ( 'NONE', #50708, .T. ) ;
#22291=EDGE_LOOP ( 'NONE', ( #36495, #34495, #39904, #43641, #26264, #49388, #11147, #40958, #32514, #26245, #23913, #50298 ) ) ;
#22327=EDGE_LOOP ( 'NONE', ( #23453, #38338, #45116, #3696, #32306 ) ) ;
#22331=LINE ( 'NONE', #2824, #10944 ) ;
#22343=LINE ( 'NONE', #26956, #37118 ) ;
#22345=LINE ( 'NONE', #30066, #21294 ) ;
#22351=DIRECTION ( 'NONE',  ( 1.000000000000000000, 0.000000000000000000, 0.000000000000000000 ) ) ;
#22353=EDGE_CURVE ( 'NONE', #14100, #11215, #15323, .T. ) ;
#22363=EDGE_CURVE ( 'NONE', #21950, #48177, #13163, .T. ) ;
#22383=DIRECTION ( 'NONE',  ( 0.000000000000000000, -0.000000000000000000, -1.000000000000000000 ) ) ;
#22388=ORIENTED_EDGE ( 'NONE', *, *, #45597, .F. ) ;
#22427=ORIENTED_EDGE ( 'NONE', *, *, #6548, .F. ) ;
#22436=DIRECTION ( 'NONE',  ( 0.000000000000000000, 1.000000000000000000, 0.000000000000000000 ) ) ;
#22444=LINE ( 'NONE', #2931, #29420 ) ;
#22447=FACE_OUTER_BOUND ( 'NONE', #1840, .T. ) ;
#22462=EDGE_CURVE ( 'NONE', #37651, #12891, #32941, .T. ) ;
#22463=CARTESIAN_POINT ( 'NONE',  ( -176.3085477938156487, -62.49999999999998579, -19.92876838486919411 ) ) ;
#22526=CARTESIAN_POINT ( 'NONE',  ( -50.00000000000000000, 0.000000000000000000, 900.0000000000000000 ) ) ;
#22527=EDGE_CURVE ( 'NONE', #40407, #15139, #26477, .T. ) ;
#22532=DIRECTION ( 'NONE',  ( -0.000000000000000000, -1.000000000000000000, -0.000000000000000000 ) ) ;
#22547=CARTESIAN_POINT ( 'NONE',  ( -178.1763882397830798, 47.50000000000000000, -120.5992382549688955 ) ) ;
#22548=CARTESIAN_POINT ( 'NONE',  ( -215.0000000000000568, 0.000000000000000000, 10.00000000000000000 ) ) ;
#22566=CARTESIAN_POINT ( 'NONE',  ( 214.9999999999999432, 164.9999999999999716, 231.9999999999999716 ) ) ;
#22603=CARTESIAN_POINT ( 'NONE',  ( -331.7552636306689351, 248.6897383013407818, 297.1446280767822259 ) ) ;
#22627=CARTESIAN_POINT ( 'NONE',  ( -225.0000000000000568, 164.9999999999999716, 111.9999999999999858 ) ) ;
#22662=VERTEX_POINT ( 'NONE', #8765 ) ;
#22667=LINE ( 'NONE', #38086, #46318 ) ;
#22675=VERTEX_POINT ( 'NONE', #28257 ) ;
#22678=EDGE_CURVE ( 'NONE', #17360, #38683, #19703, .T. ) ;
#22700=VECTOR ( 'NONE', #35247, 1000.000000000000000 ) ;
#22733=ORIENTED_EDGE ( 'NONE', *, *, #41518, .T. ) ;
#22737=ORIENTED_EDGE ( 'NONE', *, *, #8301, .T. ) ;
#22741=CARTESIAN_POINT ( 'NONE',  ( -194.9999999999999432, -172.9999999999999716, 252.0000000000000568 ) ) ;
#22751=EDGE_CURVE ( 'NONE', #37293, #26564, #34352, .T. ) ;
#22791=LINE ( 'NONE', #26895, #4015 ) ;
#22826=VECTOR ( 'NONE', #13169, 999.9999999999998863 ) ;
#22835=ORIENTED_EDGE ( 'NONE', *, *, #34901, .F. ) ;
#22840=LINE ( 'NONE', #6684, #4603 ) ;
#22842=EDGE_LOOP ( 'NONE', ( #19534, #35082, #43134, #42720, #8089, #36965, #29934, #22427, #42295, #45580 ) ) ;
#22843=EDGE_LOOP ( 'NONE', ( #40284, #48260, #10305, #8285, #18506, #23237, #24142, #19951, #49884, #28921, #44172, #50625, #27349, #45535, #29777, #40674, #15396, #35871, #34571, #17298, #4939, #39554, #13209, #11113, #30948, #44409, #24612, #47008, #9288, #3345 ) ) ;
#22885=DIRECTION ( 'NONE',  ( 0.8637789008984335659, -0.000000000000000000, 0.5038710255240859137 ) ) ;
#22888=CARTESIAN_POINT ( 'NONE',  ( 224.9999999999999432, -175.0000000000000000, 500.0000000000000000 ) ) ;
#22895=AXIS2_PLACEMENT_3D ( 'NONE', #36556, #4969, #24234 ) ;
#22902=CARTESIAN_POINT ( 'NONE',  ( -214.9999999999999432, 173.0000000000000000, 372.0000000000000000 ) ) ;
#22905=ORIENTED_EDGE ( 'NONE', *, *, #4223, .F. ) ;
#22945=VECTOR ( 'NONE', #3081, 1000.000000000000000 ) ;
#22960=AXIS2_PLACEMENT_3D ( 'NONE', #37563, #6735, #22383 ) ;
#22966=ORIENTED_EDGE ( 'NONE', *, *, #3261, .F. ) ;
#22971=STYLED_ITEM('',(#50754),#5950);
#22974=VERTEX_POINT ( 'NONE', #39217 ) ;
#22977=DIRECTION ( 'NONE',  ( 0.000000000000000000, -0.4436251537532894806, 0.8962124318248270161 ) ) ;
#22983=VERTEX_POINT ( 'NONE', #30754 ) ;
#22984=ORIENTED_EDGE ( 'NONE', *, *, #31343, .F. ) ;
#22987=CARTESIAN_POINT ( 'NONE',  ( -49.99999999999999289, 0.000000000000000000, 800.0000000000000000 ) ) ;
#23027=DIRECTION ( 'NONE',  ( 0.000000000000000000, 0.000000000000000000, 1.000000000000000000 ) ) ;
#23069=VECTOR ( 'NONE', #4516, 1000.000000000000000 ) ;
#23081=PLANE ( 'NONE',  #16738 ) ;
#23092=CARTESIAN_POINT ( 'NONE',  ( -215.0000000000000568, 164.9999999999999716, 500.0000000000000000 ) ) ;
#23093=DIRECTION ( 'NONE',  ( -0.9928768384869219865, 0.000000000000000000, -0.1191452206184307611 ) ) ;
#23119=CARTESIAN_POINT ( 'NONE',  ( 0.000000000000000000, 0.000000000000000000, 800.0000000000000000 ) ) ;
#23141=CARTESIAN_POINT ( 'NONE',  ( 0.000000000000000000, 0.000000000000000000, 800.0000000000000000 ) ) ;
#23173=VECTOR ( 'NONE', #20583, 999.9999999999998863 ) ;
#23204=ORIENTED_EDGE ( 'NONE', *, *, #21086, .T. ) ;
#23216=ORIENTED_EDGE ( 'NONE', *, *, #2631, .F. ) ;
#23222=ORIENTED_EDGE ( 'NONE', *, *, #49914, .T. ) ;
#23225=VERTEX_POINT ( 'NONE', #30432 ) ;
#23237=ORIENTED_EDGE ( 'NONE', *, *, #14934, .F. ) ;
#23266=DIRECTION ( 'NONE',  ( 0.000000000000000000, 0.000000000000000000, 1.000000000000000000 ) ) ;
#23269=ORIENTED_EDGE ( 'NONE', *, *, #718, .T. ) ;
#23300=PRODUCT_DEFINITION_SHAPE ( 'NONE', 'NONE',  #13035 ) ;
#23357=CARTESIAN_POINT ( 'NONE',  ( -177.4999999999999716, 112.5000000000000000, -10.00000000000000000 ) ) ;
#23372=EDGE_CURVE ( 'NONE', #30042, #43155, #20034, .T. ) ;
#23375=DIRECTION ( 'NONE',  ( 0.4436251537532894806, 0.000000000000000000, -0.8962124318248270161 ) ) ;
#23406=VECTOR ( 'NONE', #3047, 1000.000000000000000 ) ;
#23413=VECTOR ( 'NONE', #17156, 1000.000000000000114 ) ;
#23448=DIRECTION ( 'NONE',  ( 0.000000000000000000, 1.000000000000000000, -1.822804496942679766E-16 ) ) ;
#23453=ORIENTED_EDGE ( 'NONE', *, *, #18181, .T. ) ;
#23462=EDGE_LOOP ( 'NONE', ( #50514, #6762, #29120 ) ) ;
#23463=ORIENTED_EDGE ( 'NONE', *, *, #3581, .T. ) ;
#23464=CARTESIAN_POINT ( 'NONE',  ( 0.000000000000000000, 0.000000000000000000, 900.0000000000000000 ) ) ;
#23478=EDGE_CURVE ( 'NONE', #16604, #6362, #25451, .T. ) ;
#23480=ORIENTED_EDGE ( 'NONE', *, *, #32954, .T. ) ;
#23505=CARTESIAN_POINT ( 'NONE',  ( -239.0000000000000853, -165.6999999999999602, 250.3600000000000136 ) ) ;
#23506=AXIS2_PLACEMENT_3D ( 'NONE', #21715, #17367, #9917 ) ;
#23510=ORIENTED_EDGE ( 'NONE', *, *, #6186, .T. ) ;
#23532=VERTEX_POINT ( 'NONE', #11315 ) ;
#23551=ORIENTED_EDGE ( 'NONE', *, *, #3949, .F. ) ;
#23591=DIRECTION ( 'NONE',  ( 0.000000000000000000, 0.000000000000000000, 1.000000000000000000 ) ) ;
#23597=EDGE_LOOP ( 'NONE', ( #49938, #11811, #5852 ) ) ;
#23607=LINE ( 'NONE', #23357, #13433 ) ;
#23626=DIRECTION ( 'NONE',  ( 0.000000000000000000, -1.000000000000000000, 0.000000000000000000 ) ) ;
#23685=CIRCLE ( 'NONE', #30230, 3.500000000000003109 ) ;
#23715=PLANE ( 'NONE',  #5054 ) ;
#23719=FACE_OUTER_BOUND ( 'NONE', #50582, .T. ) ;
#23724=CIRCLE ( 'NONE', #17945, 50.00000000000000000 ) ;
#23727=ORIENTED_EDGE ( 'NONE', *, *, #22678, .F. ) ;
#23734=ORIENTED_EDGE ( 'NONE', *, *, #24654, .F. ) ;
#23739=ORIENTED_EDGE ( 'NONE', *, *, #28962, .T. ) ;
#23741=DIRECTION ( 'NONE',  ( 0.000000000000000000, -1.000000000000000000, 8.021842663476564905E-17 ) ) ;
#23748=EDGE_CURVE ( 'NONE', #12164, #23225, #7984, .T. ) ;
#23763=LINE ( 'NONE', #15042, #7914 ) ;
#23783=CARTESIAN_POINT ( 'NONE',  ( 167.5000000000000000, 102.5000000000000142, 10.00000000000000000 ) ) ;
#23790=ORIENTED_EDGE ( 'NONE', *, *, #31606, .T. ) ;
#23823=DIRECTION ( 'NONE',  ( -1.000000000000000000, -0.000000000000000000, -0.000000000000000000 ) ) ;
#23851=ORIENTED_EDGE ( 'NONE', *, *, #28462, .T. ) ;
#23854=CARTESIAN_POINT ( 'NONE',  ( -0.5000000000000000000, 0.5000000000000000000, 1000.000000000000000 ) ) ;
#23885=ORIENTED_EDGE ( 'NONE', *, *, #16405, .F. ) ;
#23888=VECTOR ( 'NONE', #3565, 1000.000000000000000 ) ;
#23892=ORIENTED_EDGE ( 'NONE', *, *, #9042, .T. ) ;
#23900=CARTESIAN_POINT ( 'NONE',  ( 224.9999999999999716, -164.9999999999999716, 444.9999999999998295 ) ) ;
#23906=EDGE_LOOP ( 'NONE', ( #2299, #18276, #50072 ) ) ;
#23907=DIRECTION ( 'NONE',  ( 0.000000000000000000, 0.000000000000000000, 1.000000000000000000 ) ) ;
#23913=ORIENTED_EDGE ( 'NONE', *, *, #5449, .F. ) ;
#23915=LINE ( 'NONE', #4169, #8928 ) ;
#23945=LINE ( 'NONE', #3419, #39441 ) ;
#23959=DIRECTION ( 'NONE',  ( -0.4055129968046615185, 0.4055129968046615185, -0.8192181753629523833 ) ) ;
#23989=LINE ( 'NONE', #11938, #35749 ) ;
#24002=ORIENTED_EDGE ( 'NONE', *, *, #22363, .F. ) ;
#24003=VECTOR ( 'NONE', #2739, 1000.000000000000000 ) ;
#24018=ADVANCED_BREP_SHAPE_REPRESENTATION ( '', ( #5950, #45486 ), #11091 ) ;
#24022=ORIENTED_EDGE ( 'NONE', *, *, #15278, .T. ) ;
#24023=DIRECTION ( 'NONE',  ( 0.000000000000000000, -0.9230769230769231282, 0.3846153846153845812 ) ) ;
#24041=EDGE_CURVE ( 'NONE', #14784, #2021, #11764, .T. ) ;
#24060=FACE_OUTER_BOUND ( 'NONE', #11396, .T. ) ;
#24097=FACE_OUTER_BOUND ( 'NONE', #33409, .T. ) ;
#24101=ADVANCED_FACE ( 'NONE', ( #19957 ), #480, .F. ) ;
#24105=CARTESIAN_POINT ( 'NONE',  ( -177.4999999999999716, -112.5000000000000000, -10.00000000000000000 ) ) ;
#24106=ADVANCED_FACE ( 'NONE', ( #38718 ), #34878, .F. ) ;
#24107=DIRECTION ( 'NONE',  ( 0.000000000000000000, 1.000000000000000000, 0.000000000000000000 ) ) ;
#24112=EDGE_CURVE ( 'NONE', #11165, #26268, #43049, .T. ) ;
#24119=DIRECTION ( 'NONE',  ( -0.4740998230350175202, -0.3386427307392980701, -0.8127425537743157014 ) ) ;
#24122=DIRECTION ( 'NONE',  ( 1.000000000000000000, 0.000000000000000000, 0.000000000000000000 ) ) ;
#24124=ORIENTED_EDGE ( 'NONE', *, *, #28791, .T. ) ;
#24131=ORIENTED_EDGE ( 'NONE', *, *, #26022, .T. ) ;
#24134=CARTESIAN_POINT ( 'NONE',  ( 214.9999999999999432, -172.9999999999999716, 252.0000000000000000 ) ) ;
#24136=ORIENTED_EDGE ( 'NONE', *, *, #36339, .T. ) ;
#24141=LINE ( 'NONE', #19766, #44959 ) ;
#24142=ORIENTED_EDGE ( 'NONE', *, *, #18298, .T. ) ;
#24145=VERTEX_POINT ( 'NONE', #38976 ) ;
#24146=EDGE_CURVE ( 'NONE', #32176, #30532, #8175, .T. ) ;
#24151=ORIENTED_EDGE ( 'NONE', *, *, #9273, .F. ) ;
#24155=AXIS2_PLACEMENT_3D ( 'NONE', #35107, #50681, #31758 ) ;
#24173=ORIENTED_EDGE ( 'NONE', *, *, #45696, .T. ) ;
#24204=VECTOR ( 'NONE', #14559, 1000.000000000000000 ) ;
#24210=VECTOR ( 'NONE', #17518, 1000.000000000000000 ) ;
#24233=PLANE ( 'NONE',  #11773 ) ;
#24234=DIRECTION ( 'NONE',  ( 1.000000000000000000, 0.000000000000000000, 0.000000000000000000 ) ) ;
#24242=DIRECTION ( 'NONE',  ( 1.000000000000000000, 0.000000000000000000, 0.000000000000000000 ) ) ;
#24302=DIRECTION ( 'NONE',  ( -0.000000000000000000, 0.000000000000000000, 1.000000000000000000 ) ) ;
#24311=DIRECTION ( 'NONE',  ( 0.1346615698592613930, 0.000000000000000000, -0.9908916497796513845 ) ) ;
#24329=LINE ( 'NONE', #13249, #18507 ) ;
#24357=EDGE_CURVE ( 'NONE', #49308, #5026, #6337, .T. ) ;
#24371=LINE ( 'NONE', #759, #29281 ) ;
#24373=CARTESIAN_POINT ( 'NONE',  ( -567.5000000000000000, -72.50000000000001421, -183.5999999999997954 ) ) ;
#24374=ORIENTED_EDGE ( 'NONE', *, *, #49096, .T. ) ;
#24388=ORIENTED_EDGE ( 'NONE', *, *, #27165, .F. ) ;
#24396=ADVANCED_FACE ( 'NONE', ( #29431 ), #29940, .F. ) ;
#24423=DIRECTION ( 'NONE',  ( -0.000000000000000000, -0.000000000000000000, 1.000000000000000000 ) ) ;
#24429=DIRECTION ( 'NONE',  ( 0.000000000000000000, -0.000000000000000000, -1.000000000000000000 ) ) ;
#24443=ORIENTED_EDGE ( 'NONE', *, *, #42945, .F. ) ;
#24446=ORIENTED_EDGE ( 'NONE', *, *, #3326, .F. ) ;
#24448=ADVANCED_FACE ( 'NONE', ( #34821 ), #11699, .F. ) ;
#24460=VECTOR ( 'NONE', #33684, 1000.000000000000000 ) ;
#24466=CARTESIAN_POINT ( 'NONE',  ( -167.4999999999999432, 47.50000000000000000, -120.5992382549688955 ) ) ;
#24494=CARTESIAN_POINT ( 'NONE',  ( 194.9999999999999432, -173.0000000000000000, 352.0000000000000568 ) ) ;
#24521=VERTEX_POINT ( 'NONE', #15043 ) ;
#24531=CARTESIAN_POINT ( 'NONE',  ( 177.5000000000000284, -112.5000000000000000, -10.00000000000000000 ) ) ;
#24548=ORIENTED_EDGE ( 'NONE', *, *, #48422, .T. ) ;
#24553=CARTESIAN_POINT ( 'NONE',  ( -194.9999999999999432, -173.0000000000000000, 352.0000000000000568 ) ) ;
#24590=DIRECTION ( 'NONE',  ( 0.000000000000000000, -1.000000000000000000, 0.000000000000000000 ) ) ;
#24600=VECTOR ( 'NONE', #43566, 1000.000000000000000 ) ;
#24612=ORIENTED_EDGE ( 'NONE', *, *, #5533, .F. ) ;
#24622=ORIENTED_EDGE ( 'NONE', *, *, #27365, .T. ) ;
#24632=EDGE_CURVE ( 'NONE', #14100, #3211, #13461, .T. ) ;
#24638=DIRECTION ( 'NONE',  ( 0.000000000000000000, -0.3846153846153844702, 0.9230769230769231282 ) ) ;
#24654=EDGE_CURVE ( 'NONE', #41260, #29654, #5260, .T. ) ;
#24673=VERTEX_POINT ( 'NONE', #49070 ) ;
#24674=DIRECTION ( 'NONE',  ( -0.000000000000000000, 2.406552799042969348E-16, 1.000000000000000000 ) ) ;
#24711=VERTEX_POINT ( 'NONE', #21664 ) ;
#24750=LINE ( 'NONE', #20122, #14763 ) ;
#24763=LINE ( 'NONE', #35560, #5429 ) ;
#24772=VECTOR ( 'NONE', #13265, 1000.000000000000000 ) ;
#24798=ORIENTED_EDGE ( 'NONE', *, *, #37324, .T. ) ;
#24817=ORIENTED_EDGE ( 'NONE', *, *, #17139, .F. ) ;
#24840=CARTESIAN_POINT ( 'NONE',  ( 50.00000000000000000, 6.123233995736766085E-15, 900.0000000000000000 ) ) ;
#24909=LINE ( 'NONE', #20546, #5366 ) ;
#24917=CARTESIAN_POINT ( 'NONE',  ( 224.9999999999999432, -175.0000000000000000, 500.0000000000000000 ) ) ;
#24928=ORIENTED_EDGE ( 'NONE', *, *, #5008, .T. ) ;
#24937=ORIENTED_EDGE ( 'NONE', *, *, #2640, .F. ) ;
#24942=FACE_BOUND ( 'NONE', #45143, .T. ) ;
#24969=ADVANCED_FACE ( 'NONE', ( #36531 ), #20598, .T. ) ;
#24970=DIRECTION ( 'NONE',  ( 0.000000000000000000, -0.9230769230769231282, 0.3846153846153845812 ) ) ;
#24983=VERTEX_POINT ( 'NONE', #24466 ) ;
#24990=FACE_BOUND ( 'NONE', #31776, .T. ) ;
#25018=LINE ( 'NONE', #29365, #21641 ) ;
#25021=EDGE_CURVE ( 'NONE', #48417, #20358, #36022, .T. ) ;
#25022=VERTEX_POINT ( 'NONE', #12895 ) ;
#25023=VECTOR ( 'NONE', #5320, 1000.000000000000000 ) ;
#25037=DIRECTION ( 'NONE',  ( -1.000000000000000000, 0.000000000000000000, -0.000000000000000000 ) ) ;
#25095=CARTESIAN_POINT ( 'NONE',  ( 194.9999999999999432, 0.000000000000000000, 0.000000000000000000 ) ) ;
#25106=CARTESIAN_POINT ( 'NONE',  ( 194.9999999999999432, -173.0000000000000000, 372.0000000000000568 ) ) ;
#25149=DIRECTION ( 'NONE',  ( 0.000000000000000000, -1.000000000000000000, 0.000000000000000000 ) ) ;
#25158=ORIENTED_EDGE ( 'NONE', *, *, #38112, .T. ) ;
#25171=CARTESIAN_POINT ( 'NONE',  ( 214.9999999999999432, 164.9999999999999716, 500.0000000000000000 ) ) ;
#25181=CARTESIAN_POINT ( 'NONE',  ( 214.9999999999999432, -175.0000000000000000, 474.0000000000000000 ) ) ;
#25318=VECTOR ( 'NONE', #27879, 1000.000000000000000 ) ;
#25338=LINE ( 'NONE', #10191, #30446 ) ;
#25355=EDGE_CURVE ( 'NONE', #23532, #7894, #48886, .T. ) ;
#25367=VERTEX_POINT ( 'NONE', #44309 ) ;
#25409=CARTESIAN_POINT ( 'NONE',  ( 194.9999999999999432, -173.0000000000000000, 132.0000000000000853 ) ) ;
#25445=ORIENTED_EDGE ( 'NONE', *, *, #25570, .F. ) ;
#25451=LINE ( 'NONE', #29302, #50450 ) ;
#25455=DIRECTION ( 'NONE',  ( -1.000000000000000000, -0.000000000000000000, -0.000000000000000000 ) ) ;
#25461=DIRECTION ( 'NONE',  ( 1.000000000000000000, 0.000000000000000000, 0.000000000000000000 ) ) ;
#25465=DIRECTION ( 'NONE',  ( -1.000000000000000000, -0.000000000000000000, -0.000000000000000000 ) ) ;
#25469=DIRECTION ( 'NONE',  ( 0.000000000000000000, -0.000000000000000000, 1.000000000000000000 ) ) ;
#25475=ORIENTED_EDGE ( 'NONE', *, *, #41238, .T. ) ;
#25477=CARTESIAN_POINT ( 'NONE',  ( 194.9999999999999432, -172.9999999999999716, 232.0000000000000284 ) ) ;
#25478=VECTOR ( 'NONE', #2448, 1000.000000000000000 ) ;
#25520=ORIENTED_EDGE ( 'NONE', *, *, #49096, .F. ) ;
#25530=LINE ( 'NONE', #26543, #35654 ) ;
#25540=CARTESIAN_POINT ( 'NONE',  ( -177.4999999999999716, -72.50000000000001421, -9.999999999999973355 ) ) ;
#25546=DIRECTION ( 'NONE',  ( -1.000000000000000000, 0.000000000000000000, -0.000000000000000000 ) ) ;
#25570=EDGE_CURVE ( 'NONE', #30113, #17360, #31227, .T. ) ;
#25604=ORIENTED_EDGE ( 'NONE', *, *, #6325, .F. ) ;
#25623=ORIENTED_EDGE ( 'NONE', *, *, #8632, .T. ) ;
#25630=ORIENTED_EDGE ( 'NONE', *, *, #43141, .T. ) ;
#25643=ORIENTED_EDGE ( 'NONE', *, *, #29415, .F. ) ;
#25644=ORIENTED_EDGE ( 'NONE', *, *, #40091, .F. ) ;
#25681=VECTOR ( 'NONE', #30214, 1000.000000000000000 ) ;
#25721=VECTOR ( 'NONE', #39518, 1000.000000000000227 ) ;
#25722=CARTESIAN_POINT ( 'NONE',  ( -194.9999999999999432, 173.0000000000000000, 231.9999999999999716 ) ) ;
#25746=PLANE ( 'NONE',  #20601 ) ;
#25749=AXIS2_PLACEMENT_3D ( 'NONE', #41337, #29534, #9773 ) ;
#25780=DIRECTION ( 'NONE',  ( 0.000000000000000000, 0.000000000000000000, -1.000000000000000000 ) ) ;
#25783=CARTESIAN_POINT ( 'NONE',  ( -214.9999999999999432, 173.0000000000000000, 132.0000000000000000 ) ) ;
#25789=EDGE_CURVE ( 'NONE', #20648, #16490, #25530, .T. ) ;
#25805=VECTOR ( 'NONE', #9960, 1000.000000000000000 ) ;
#25833=FACE_OUTER_BOUND ( 'NONE', #46266, .T. ) ;
#25844=EDGE_CURVE ( 'NONE', #20358, #18930, #41433, .T. ) ;
#25902=VECTOR ( 'NONE', #25461, 1000.000000000000000 ) ;
#25916=LINE ( 'NONE', #41299, #12221 ) ;
#25927=ORIENTED_EDGE ( 'NONE', *, *, #41518, .F. ) ;
#25977=DIRECTION ( 'NONE',  ( -0.000000000000000000, -1.000000000000000000, -0.000000000000000000 ) ) ;
#25981=CARTESIAN_POINT ( 'NONE',  ( -167.4999999999999432, 47.50000000000000000, -18.87174264961130987 ) ) ;
#25983=FACE_OUTER_BOUND ( 'NONE', #33485, .T. ) ;
#25998=ORIENTED_EDGE ( 'NONE', *, *, #16899, .T. ) ;
#26008=LINE ( 'NONE', #37327, #26175 ) ;
#26014=EDGE_CURVE ( 'NONE', #33295, #44965, #40628, .T. ) ;
#26022=EDGE_CURVE ( 'NONE', #18930, #12164, #8822, .T. ) ;
#26024=CARTESIAN_POINT ( 'NONE',  ( -177.4999999999999716, 57.49999999999996447, -9.999999999999973355 ) ) ;
#26041=DIRECTION ( 'NONE',  ( 0.000000000000000000, 0.000000000000000000, 1.000000000000000000 ) ) ;
#26051=CARTESIAN_POINT ( 'NONE',  ( -33.89193117067290473, 21.24469349090191983, 910.0000000000000000 ) ) ;
#26056=CIRCLE ( 'NONE', #31826, 3.500000000000003109 ) ;
#26061=ORIENTED_EDGE ( 'NONE', *, *, #9943, .T. ) ;
#26085=CARTESIAN_POINT ( 'NONE',  ( 224.9999999999998863, -0.000000000000000000, 500.0000000000000000 ) ) ;
#26117=CARTESIAN_POINT ( 'NONE',  ( 167.5000000000000000, 102.5000000000000284, -10.00000000000000000 ) ) ;
#26126=EDGE_LOOP ( 'NONE', ( #14354, #33921, #23892, #40537 ) ) ;
#26138=ORIENTED_EDGE ( 'NONE', *, *, #18452, .T. ) ;
#26157=VECTOR ( 'NONE', #15330, 1000.000000000000000 ) ;
#26166=ORIENTED_EDGE ( 'NONE', *, *, #8750, .T. ) ;
#26175=VECTOR ( 'NONE', #26502, 1000.000000000000000 ) ;
#26178=ORIENTED_EDGE ( 'NONE', *, *, #12499, .F. ) ;
#26186=ORIENTED_EDGE ( 'NONE', *, *, #20272, .F. ) ;
#26196=ORIENTED_EDGE ( 'NONE', *, *, #39677, .T. ) ;
#26243=AXIS2_PLACEMENT_3D ( 'NONE', #48722, #32121, #24429 ) ;
#26245=ORIENTED_EDGE ( 'NONE', *, *, #20609, .F. ) ;
#26259=ORIENTED_EDGE ( 'NONE', *, *, #23478, .T. ) ;
#26264=ORIENTED_EDGE ( 'NONE', *, *, #26386, .F. ) ;
#26268=VERTEX_POINT ( 'NONE', #11594 ) ;
#26290=DIRECTION ( 'NONE',  ( 0.000000000000000000, 1.000000000000000000, 0.000000000000000000 ) ) ;
#26319=AXIS2_PLACEMENT_3D ( 'NONE', #38942, #39697, #682 ) ;
#26349=DIRECTION ( 'NONE',  ( -0.000000000000000000, -0.000000000000000000, -1.000000000000000000 ) ) ;
#26350=CARTESIAN_POINT ( 'NONE',  ( -50.00000000000000000, -50.00000000000000000, 900.0000000000000000 ) ) ;
#26369=EDGE_LOOP ( 'NONE', ( #47319, #8095, #35550, #10347, #13327 ) ) ;
#26379=ORIENTED_EDGE ( 'NONE', *, *, #42565, .T. ) ;
#26386=EDGE_CURVE ( 'NONE', #36764, #38992, #17659, .T. ) ;
#26387=DIRECTION ( 'NONE',  ( 0.000000000000000000, 0.000000000000000000, 1.000000000000000000 ) ) ;
#26396=ORIENTED_EDGE ( 'NONE', *, *, #41736, .T. ) ;
#26401=LINE ( 'NONE', #22548, #23406 ) ;
#26403=VECTOR ( 'NONE', #37849, 1000.000000000000000 ) ;
#26439=AXIS2_PLACEMENT_3D ( 'NONE', #37420, #21482, #37172 ) ;
#26448=EDGE_CURVE ( 'NONE', #35388, #27665, #45330, .T. ) ;
#26473=CARTESIAN_POINT ( 'NONE',  ( -176.3085477938156487, 57.49999999999996447, -19.92876838486919411 ) ) ;
#26477=LINE ( 'NONE', #22627, #43055 ) ;
#26482=CARTESIAN_POINT ( 'NONE',  ( 214.9999999999999432, 173.0000000000000000, 132.0000000000000000 ) ) ;
#26502=DIRECTION ( 'NONE',  ( 1.000000000000000000, 0.000000000000000000, 0.000000000000000000 ) ) ;
#26507=DIRECTION ( 'NONE',  ( 0.000000000000000000, -0.000000000000000000, 1.000000000000000000 ) ) ;
#26518=EDGE_CURVE ( 'NONE', #26564, #6437, #14818, .T. ) ;
#26524=EDGE_CURVE ( 'NONE', #5061, #1180, #50323, .T. ) ;
#26538=DIRECTION ( 'NONE',  ( 0.000000000000000000, 1.000000000000000000, -2.406552799042969348E-16 ) ) ;
#26542=EDGE_CURVE ( 'NONE', #19082, #1605, #35108, .T. ) ;
#26543=CARTESIAN_POINT ( 'NONE',  ( 214.9999999999999432, -173.0000000000000000, 352.0000000000000568 ) ) ;
#26564=VERTEX_POINT ( 'NONE', #15837 ) ;
#26581=EDGE_CURVE ( 'NONE', #34586, #24521, #3507, .T. ) ;
#26587=PLANE ( 'NONE',  #47445 ) ;
#26601=CARTESIAN_POINT ( 'NONE',  ( 232.4999999999999716, -169.9999999999999716, 4.999999999999616307 ) ) ;
#26613=DIRECTION ( 'NONE',  ( -1.000000000000000000, 0.000000000000000000, 0.000000000000000000 ) ) ;
#26650=CARTESIAN_POINT ( 'NONE',  ( -582.5000000000000000, 57.49999999999996447, -58.60000000000003695 ) ) ;
#26700=VECTOR ( 'NONE', #12150, 1000.000000000000000 ) ;
#26705=ORIENTED_EDGE ( 'NONE', *, *, #14056, .T. ) ;
#26713=DIRECTION ( 'NONE',  ( 0.000000000000000000, 0.000000000000000000, 1.000000000000000000 ) ) ;
#26715=ORIENTED_EDGE ( 'NONE', *, *, #32744, .T. ) ;
#26731=VERTEX_POINT ( 'NONE', #17096 ) ;
#26755=AXIS2_PLACEMENT_3D ( 'NONE', #6203, #41092, #36513 ) ;
#26756=DIRECTION ( 'NONE',  ( -0.000000000000000000, -0.2791762785758810095, 0.9602398687205827565 ) ) ;
#26776=ORIENTED_EDGE ( 'NONE', *, *, #25021, .F. ) ;
#26804=CARTESIAN_POINT ( 'NONE',  ( 232.4999999999999716, -169.9999999999999716, 32.29650858650035161 ) ) ;
#26807=ADVANCED_FACE ( 'NONE', ( #35864 ), #43782, .T. ) ;
#26809=DIRECTION ( 'NONE',  ( 1.000000000000000000, 0.000000000000000000, 0.000000000000000000 ) ) ;
#26813=LINE ( 'NONE', #49348, #10630 ) ;
#26817=DIRECTION ( 'NONE',  ( 0.000000000000000000, 0.000000000000000000, -1.000000000000000000 ) ) ;
#26855=DIRECTION ( 'NONE',  ( 0.000000000000000000, -0.3846153846153845812, -0.9230769230769231282 ) ) ;
#26885=PLANE ( 'NONE',  #15900 ) ;
#26895=CARTESIAN_POINT ( 'NONE',  ( -194.9999999999999432, 164.9999999999999716, 500.0000000000000000 ) ) ;
#26915=LINE ( 'NONE', #27180, #1949 ) ;
#26916=DIRECTION ( 'NONE',  ( -0.4740998230350175202, 0.3386427307392980701, -0.8127425537743157014 ) ) ;
#26939=EDGE_CURVE ( 'NONE', #27665, #41907, #41957, .T. ) ;
#26956=CARTESIAN_POINT ( 'NONE',  ( -214.9999999999999432, -172.9999999999999716, 232.0000000000000284 ) ) ;
#26968=VECTOR ( 'NONE', #43636, 1000.000000000000000 ) ;
#26972=VECTOR ( 'NONE', #28234, 1000.000000000000000 ) ;
#27002=CARTESIAN_POINT ( 'NONE',  ( 432.7825420346616170, 74.83106485270648989, -120.5992382549688955 ) ) ;
#27009=LINE ( 'NONE', #22902, #11115 ) ;
#27020=ORIENTED_EDGE ( 'NONE', *, *, #26448, .F. ) ;
#27027=ORIENTED_EDGE ( 'NONE', *, *, #13758, .T. ) ;
#27057=EDGE_CURVE ( 'NONE', #33060, #4645, #3191, .T. ) ;
#27080=CARTESIAN_POINT ( 'NONE',  ( 194.9999999999999432, -173.0000000000000000, 132.0000000000000853 ) ) ;
#27086=( GEOMETRIC_REPRESENTATION_CONTEXT ( 3 ) GLOBAL_UNCERTAINTY_ASSIGNED_CONTEXT ( ( #16902 ) ) GLOBAL_UNIT_ASSIGNED_CONTEXT ( ( #2311, #50216, #49475 ) ) REPRESENTATION_CONTEXT ( 'NONE', 'WORKASPACE' ) );
#27099=CARTESIAN_POINT ( 'NONE',  ( -194.9999999999999432, -173.0000000000000000, 372.0000000000000568 ) ) ;
#27137=CARTESIAN_POINT ( 'NONE',  ( 0.000000000000000000, 0.000000000000000000, 910.0000000000000000 ) ) ;
#27150=VECTOR ( 'NONE', #40613, 1000.000000000000000 ) ;
#27165=EDGE_CURVE ( 'NONE', #41907, #22974, #21136, .T. ) ;
#27180=CARTESIAN_POINT ( 'NONE',  ( 177.5000000000000284, -102.5000000000000142, -8.575805527524005711 ) ) ;
#27209=LINE ( 'NONE', #23092, #13921 ) ;
#27212=EDGE_LOOP ( 'NONE', ( #27846, #32581, #15855, #21923 ) ) ;
#27214=LINE ( 'NONE', #43607, #17403 ) ;
#27232=CARTESIAN_POINT ( 'NONE',  ( 397.9839762253770346, 0.000000000000000000, 197.0020682315616796 ) ) ;
#27237=DIRECTION ( 'NONE',  ( 0.000000000000000000, 0.000000000000000000, -1.000000000000000000 ) ) ;
#27248=EDGE_LOOP ( 'NONE', ( #7022, #3920, #23885, #34807 ) ) ;
#27250=VECTOR ( 'NONE', #37341, 1000.000000000000000 ) ;
#27267=DIRECTION ( 'NONE',  ( 0.000000000000000000, 1.000000000000000000, -1.822804496942679766E-16 ) ) ;
#27269=LINE ( 'NONE', #2634, #12312 ) ;
#27271=FACE_OUTER_BOUND ( 'NONE', #9727, .T. ) ;
#27282=FACE_BOUND ( 'NONE', #8061, .T. ) ;
#27283=VERTEX_POINT ( 'NONE', #19047 ) ;
#27292=ORIENTED_EDGE ( 'NONE', *, *, #15196, .F. ) ;
#27349=ORIENTED_EDGE ( 'NONE', *, *, #16309, .T. ) ;
#27357=CARTESIAN_POINT ( 'NONE',  ( 0.000000000000000000, 0.000000000000000000, 800.0000000000000000 ) ) ;
#27365=EDGE_CURVE ( 'NONE', #44977, #35508, #27009, .T. ) ;
#27368=LINE ( 'NONE', #35348, #41655 ) ;
#27443=ADVANCED_FACE ( 'NONE', ( #39337 ), #35998, .F. ) ;
#27448=CARTESIAN_POINT ( 'NONE',  ( 44.25629667545849344, 0.000000000000000000, 790.0000000000000000 ) ) ;
#27449=ORIENTED_EDGE ( 'NONE', *, *, #13638, .T. ) ;
#27456=CARTESIAN_POINT ( 'NONE',  ( -331.7552636306689919, -248.6897383013407250, 297.1446280767822259 ) ) ;
#27486=ORIENTED_EDGE ( 'NONE', *, *, #37740, .T. ) ;
#27515=ORIENTED_EDGE ( 'NONE', *, *, #40862, .T. ) ;
#27522=VERTEX_POINT ( 'NONE', #5424 ) ;
#27532=PLANE ( 'NONE',  #15594 ) ;
#27556=CARTESIAN_POINT ( 'NONE',  ( -7.884183412771427868, -42.26678417219198991, 893.0811050474360400 ) ) ;
#27566=( NAMED_UNIT ( * ) PLANE_ANGLE_UNIT ( ) SI_UNIT ( $, .RADIAN. ) );
#27583=ORIENTED_EDGE ( 'NONE', *, *, #36339, .F. ) ;
#27613=CARTESIAN_POINT ( 'NONE',  ( 40.00000000000000000, 7.564790863224921225, 897.6604670114604687 ) ) ;
#27614=DIRECTION ( 'NONE',  ( 0.000000000000000000, 0.000000000000000000, -1.000000000000000000 ) ) ;
#27665=VERTEX_POINT ( 'NONE', #3592 ) ;
#27683=DIRECTION ( 'NONE',  ( -0.1191452206184307749, 0.000000000000000000, 0.9928768384869220975 ) ) ;
#27691=AXIS2_PLACEMENT_3D ( 'NONE', #30651, #26290, #45500 ) ;
#27702=EDGE_CURVE ( 'NONE', #31054, #48005, #45908, .T. ) ;
#27707=EDGE_CURVE ( 'NONE', #41718, #44615, #22840, .T. ) ;
#27790=CARTESIAN_POINT ( 'NONE',  ( 240.0000000000000000, -164.9999999999999716, 444.9999999999998295 ) ) ;
#27804=EDGE_LOOP ( 'NONE', ( #38017, #39969, #38834, #13911 ) ) ;
#27814=CARTESIAN_POINT ( 'NONE',  ( -0.5000000000000000000, 0.5000000000000000000, 1000.000000000000000 ) ) ;
#27846=ORIENTED_EDGE ( 'NONE', *, *, #19605, .F. ) ;
#27879=DIRECTION ( 'NONE',  ( 0.000000000000000000, 0.2791762785758810650, -0.9602398687205827565 ) ) ;
#27907=CARTESIAN_POINT ( 'NONE',  ( 194.9999999999999432, -172.9999999999999716, 252.0000000000000568 ) ) ;
#27920=CARTESIAN_POINT ( 'NONE',  ( 0.000000000000000000, 0.000000000000000000, 900.0000000000000000 ) ) ;
#27929=DIRECTION ( 'NONE',  ( 0.4740998230350172427, -0.3386427307392981256, -0.8127425537743157014 ) ) ;
#27939=DIRECTION ( 'NONE',  ( 0.9928768384869219865, 0.000000000000000000, 0.1191452206184307611 ) ) ;
#27969=EDGE_LOOP ( 'NONE', ( #38945, #26705, #33332, #22966, #7954 ) ) ;
#27998=ADVANCED_FACE ( 'NONE', ( #36182 ), #37206, .T. ) ;
#28030=CARTESIAN_POINT ( 'NONE',  ( 50.00000000000000000, 50.00000000000000000, 900.0000000000000000 ) ) ;
#28046=LINE ( 'NONE', #40114, #27150 ) ;
#28068=CARTESIAN_POINT ( 'NONE',  ( 214.9999999999999432, -317.3964497041420145, 132.2485207100591253 ) ) ;
#28118=LINE ( 'NONE', #31469, #2661 ) ;
#28132=VECTOR ( 'NONE', #44830, 1000.000000000000000 ) ;
#28199=LINE ( 'NONE', #32309, #1560 ) ;
#28204=EDGE_CURVE ( 'NONE', #12891, #26731, #24763, .T. ) ;
#28206=VECTOR ( 'NONE', #13806, 1000.000000000000000 ) ;
#28214=VERTEX_POINT ( 'NONE', #4992 ) ;
#28234=DIRECTION ( 'NONE',  ( 1.000000000000000000, -0.000000000000000000, -0.000000000000000000 ) ) ;
#28240=ORIENTED_EDGE ( 'NONE', *, *, #15775, .T. ) ;
#28242=CARTESIAN_POINT ( 'NONE',  ( 224.9999999999999716, -164.9999999999999716, 474.9999999999998863 ) ) ;
#28254=SHAPE_DEFINITION_REPRESENTATION ( #23300, #15926 ) ;
#28257=CARTESIAN_POINT ( 'NONE',  ( 40.00000000000000000, 4.898587196589413026E-15, 897.6604670114603550 ) ) ;
#28260=ORIENTED_EDGE ( 'NONE', *, *, #5449, .T. ) ;
#28266=VECTOR ( 'NONE', #7130, 1000.000000000000000 ) ;
#28269=VECTOR ( 'NONE', #9755, 1000.000000000000000 ) ;
#28304=VECTOR ( 'NONE', #5213, 1000.000000000000000 ) ;
#28319=LINE ( 'NONE', #47530, #35421 ) ;
#28324=DIRECTION ( 'NONE',  ( 0.1346615698592613930, 0.000000000000000000, -0.9908916497796513845 ) ) ;
#28325=ORIENTED_EDGE ( 'NONE', *, *, #28927, .F. ) ;
#28331=VECTOR ( 'NONE', #18840, 1000.000000000000114 ) ;
#28339=AXIS2_PLACEMENT_3D ( 'NONE', #16526, #12412, #20112 ) ;
#28361=CARTESIAN_POINT ( 'NONE',  ( 0.000000000000000000, 33.89193117067290473, 910.0000000000000000 ) ) ;
#28440=LINE ( 'NONE', #16373, #12870 ) ;
#28454=ORIENTED_EDGE ( 'NONE', *, *, #5477, .T. ) ;
#28462=EDGE_CURVE ( 'NONE', #3211, #5210, #15469, .T. ) ;
#28476=LINE ( 'NONE', #47923, #14747 ) ;
#28485=DIRECTION ( 'NONE',  ( -0.000000000000000000, -0.000000000000000000, -1.000000000000000000 ) ) ;
#28496=ORIENTED_EDGE ( 'NONE', *, *, #21120, .T. ) ;
#28519=AXIS2_PLACEMENT_3D ( 'NONE', #10447, #18137, #49651 ) ;
#28542=ORIENTED_EDGE ( 'NONE', *, *, #50551, .T. ) ;
#28552=DIRECTION ( 'NONE',  ( -1.000000000000000000, 0.000000000000000000, 0.000000000000000000 ) ) ;
#28600=LINE ( 'NONE', #35567, #21773 ) ;
#28607=ORIENTED_EDGE ( 'NONE', *, *, #20609, .T. ) ;
#28617=ORIENTED_EDGE ( 'NONE', *, *, #33672, .T. ) ;
#28652=VECTOR ( 'NONE', #4228, 1000.000000000000000 ) ;
#28659=VECTOR ( 'NONE', #12829, 1000.000000000000000 ) ;
#28678=EDGE_CURVE ( 'NONE', #23532, #16113, #41474, .T. ) ;
#28684=ADVANCED_FACE ( 'NONE', ( #44904 ), #36767, .T. ) ;
#28685=CARTESIAN_POINT ( 'NONE',  ( 194.9999999999999432, 173.0000000000000000, 132.0000000000000000 ) ) ;
#28699=CARTESIAN_POINT ( 'NONE',  ( -40.00000000000000000, 0.000000000000000000, 897.6604670114603550 ) ) ;
#28713=CARTESIAN_POINT ( 'NONE',  ( -194.9999999999999432, 164.9999999999999716, 500.0000000000000000 ) ) ;
#28756=DIRECTION ( 'NONE',  ( 0.000000000000000000, -1.000000000000000000, 0.000000000000000000 ) ) ;
#28765=AXIS2_PLACEMENT_3D ( 'NONE', #15221, #11361, #26507 ) ;
#28770=ORIENTED_EDGE ( 'NONE', *, *, #31005, .F. ) ;
#28785=FACE_OUTER_BOUND ( 'NONE', #17287, .T. ) ;
#28786=ORIENTED_EDGE ( 'NONE', *, *, #21086, .F. ) ;
#28791=EDGE_CURVE ( 'NONE', #1717, #24673, #7474, .T. ) ;
#28818=FACE_OUTER_BOUND ( 'NONE', #12388, .T. ) ;
#28850=CARTESIAN_POINT ( 'NONE',  ( 228.9999999999999716, -169.9999999999999716, 32.29650858650035161 ) ) ;
#28858=CARTESIAN_POINT ( 'NONE',  ( -215.0000000000000568, -175.0000000000000000, 500.0000000000000000 ) ) ;
#28864=VERTEX_POINT ( 'NONE', #18493 ) ;
#28902=LINE ( 'NONE', #21442, #35598 ) ;
#28903=ORIENTED_EDGE ( 'NONE', *, *, #13082, .F. ) ;
#28921=ORIENTED_EDGE ( 'NONE', *, *, #44461, .F. ) ;
#28927=EDGE_CURVE ( 'NONE', #42445, #49554, #6953, .T. ) ;
#28930=DIRECTION ( 'NONE',  ( 0.000000000000000000, -0.9602398687205827565, -0.2791762785758810650 ) ) ;
#28939=DIRECTION ( 'NONE',  ( 0.000000000000000000, -1.000000000000000000, 1.604368532695312981E-16 ) ) ;
#28948=DIRECTION ( 'NONE',  ( 0.000000000000000000, 0.000000000000000000, -1.000000000000000000 ) ) ;
#28953=ORIENTED_EDGE ( 'NONE', *, *, #44640, .T. ) ;
#28962=EDGE_CURVE ( 'NONE', #26731, #32176, #1031, .T. ) ;
#28994=DIRECTION ( 'NONE',  ( 0.000000000000000000, 0.000000000000000000, -1.000000000000000000 ) ) ;
#29001=FACE_OUTER_BOUND ( 'NONE', #31573, .T. ) ;
#29020=FACE_OUTER_BOUND ( 'NONE', #7499, .T. ) ;
#29047=ADVANCED_FACE ( 'NONE', ( #36717 ), #17683, .T. ) ;
#29053=DIRECTION ( 'NONE',  ( 0.000000000000000000, 1.000000000000000000, -2.406552799042969348E-16 ) ) ;
#29081=EDGE_CURVE ( 'NONE', #15483, #44977, #32594, .T. ) ;
#29092=VECTOR ( 'NONE', #16126, 1000.000000000000000 ) ;
#29107=CARTESIAN_POINT ( 'NONE',  ( 50.00000000000000000, 50.00000000000000000, 800.0000000000000000 ) ) ;
#29117=VECTOR ( 'NONE', #23959, 1000.000000000000114 ) ;
#29120=ORIENTED_EDGE ( 'NONE', *, *, #18324, .T. ) ;
#29126=CARTESIAN_POINT ( 'NONE',  ( -40.00000000000000000, 0.000000000000000000, 900.0000000000000000 ) ) ;
#29149=VECTOR ( 'NONE', #2127, 1000.000000000000000 ) ;
#29163=AXIS2_PLACEMENT_3D ( 'NONE', #9633, #12958, #4767 ) ;
#29218=ORIENTED_EDGE ( 'NONE', *, *, #14934, .T. ) ;
#29221=EDGE_LOOP ( 'NONE', ( #39593, #28260, #4694, #40568, #25520 ) ) ;
#29222=DIRECTION ( 'NONE',  ( 0.000000000000000000, -1.000000000000000000, 1.604368532695312981E-16 ) ) ;
#29239=EDGE_LOOP ( 'NONE', ( #21061, #24002, #33720, #11432 ) ) ;
#29241=LINE ( 'NONE', #1294, #28659 ) ;
#29260=CARTESIAN_POINT ( 'NONE',  ( -33.89193117067290473, -21.24469349090191983, 910.0000000000000000 ) ) ;
#29279=EDGE_CURVE ( 'NONE', #25367, #46103, #49442, .T. ) ;
#29281=VECTOR ( 'NONE', #24122, 1000.000000000000000 ) ;
#29302=CARTESIAN_POINT ( 'NONE',  ( 214.9999999999999432, -173.0000000000000000, 112.0000000000000284 ) ) ;
#29310=DIRECTION ( 'NONE',  ( -0.8962124318248270161, 0.000000000000000000, 0.4436251537532894806 ) ) ;
#29311=CARTESIAN_POINT ( 'NONE',  ( -225.0000000000000568, 164.9999999999999716, 372.0000000000000000 ) ) ;
#29340=FACE_OUTER_BOUND ( 'NONE', #6068, .T. ) ;
#29355=AXIS2_PLACEMENT_3D ( 'NONE', #26473, #27683, #27939 ) ;
#29365=CARTESIAN_POINT ( 'NONE',  ( 224.9999999999999716, -175.0000000000000000, 62.29650858650038003 ) ) ;
#29394=LINE ( 'NONE', #5798, #15578 ) ;
#29415=EDGE_CURVE ( 'NONE', #22675, #32324, #38488, .T. ) ;
#29417=ADVANCED_FACE ( 'NONE', ( #47873, #45044 ), #32280, .T. ) ;
#29420=VECTOR ( 'NONE', #36937, 1000.000000000000000 ) ;
#29427=AXIS2_PLACEMENT_3D ( 'NONE', #16959, #35963, #16199 ) ;
#29431=FACE_OUTER_BOUND ( 'NONE', #40142, .T. ) ;
#29435=LINE ( 'NONE', #9680, #24772 ) ;
#29445=ORIENTED_EDGE ( 'NONE', *, *, #8750, .F. ) ;
#29486=ORIENTED_EDGE ( 'NONE', *, *, #14888, .T. ) ;
#29488=VERTEX_POINT ( 'NONE', #48371 ) ;
#29499=CARTESIAN_POINT ( 'NONE',  ( -40.00000000000000000, 0.000000000000000000, 897.6604670114603550 ) ) ;
#29507=LINE ( 'NONE', #21810, #6041 ) ;
#29530=CARTESIAN_POINT ( 'NONE',  ( 194.9999999999999432, 164.9999999999999716, 352.0000000000000000 ) ) ;
#29534=DIRECTION ( 'NONE',  ( 0.000000000000000000, 0.000000000000000000, -1.000000000000000000 ) ) ;
#29568=VECTOR ( 'NONE', #15074, 1000.000000000000114 ) ;
#29587=DIRECTION ( 'NONE',  ( 0.000000000000000000, 0.000000000000000000, 1.000000000000000000 ) ) ;
#29598=VECTOR ( 'NONE', #23448, 1000.000000000000000 ) ;
#29630=ORIENTED_EDGE ( 'NONE', *, *, #3960, .T. ) ;
#29654=VERTEX_POINT ( 'NONE', #23505 ) ;
#29775=LINE ( 'NONE', #9763, #16382 ) ;
#29777=ORIENTED_EDGE ( 'NONE', *, *, #21532, .T. ) ;
#29783=CARTESIAN_POINT ( 'NONE',  ( -215.0000000000000568, -165.2931214222915344, 497.2965085865002948 ) ) ;
#29800=VERTEX_POINT ( 'NONE', #29805 ) ;
#29805=CARTESIAN_POINT ( 'NONE',  ( -215.0000000000000568, -175.0000000000000000, 10.00000000000000000 ) ) ;
#29814=PLANE ( 'NONE',  #12971 ) ;
#29823=VECTOR ( 'NONE', #48141, 1000.000000000000227 ) ;
#29831=CARTESIAN_POINT ( 'NONE',  ( -194.9999999999999432, -173.0000000000000000, 112.0000000000000284 ) ) ;
#29849=VECTOR ( 'NONE', #4246, 1000.000000000000000 ) ;
#29870=ORIENTED_EDGE ( 'NONE', *, *, #453, .T. ) ;
#29883=VECTOR ( 'NONE', #26387, 1000.000000000000000 ) ;
#29933=DIRECTION ( 'NONE',  ( -0.000000000000000000, 0.8962124318248270161, 0.4436251537532894806 ) ) ;
#29934=ORIENTED_EDGE ( 'NONE', *, *, #22751, .F. ) ;
#29940=PLANE ( 'NONE',  #14388 ) ;
#29946=CARTESIAN_POINT ( 'NONE',  ( 0.000000000000000000, 0.000000000000000000, 900.0000000000000000 ) ) ;
#29955=EDGE_CURVE ( 'NONE', #48177, #14442, #24371, .T. ) ;
#29958=EDGE_CURVE ( 'NONE', #40407, #40831, #39769, .T. ) ;
#29986=VECTOR ( 'NONE', #708, 1000.000000000000000 ) ;
#30011=LINE ( 'NONE', #41792, #49958 ) ;
#30029=CIRCLE ( 'NONE', #41478, 3.500000000000003109 ) ;
#30042=VERTEX_POINT ( 'NONE', #29499 ) ;
#30044=DIRECTION ( 'NONE',  ( -1.000000000000000000, 0.000000000000000000, -0.000000000000000000 ) ) ;
#30057=VERTEX_POINT ( 'NONE', #10746 ) ;
#30063=CARTESIAN_POINT ( 'NONE',  ( 194.9999999999999432, 173.0000000000000000, 231.9999999999999716 ) ) ;
#30064=FACE_OUTER_BOUND ( 'NONE', #16477, .T. ) ;
#30066=CARTESIAN_POINT ( 'NONE',  ( 214.9999999999999432, -175.0000000000000000, 500.0000000000000000 ) ) ;
#30087=DIRECTION ( 'NONE',  ( 0.4055129968046615185, 0.4055129968046615185, -0.8192181753629524943 ) ) ;
#30094=CARTESIAN_POINT ( 'NONE',  ( 0.000000000000000000, 0.000000000000000000, 910.0000000000000000 ) ) ;
#30113=VERTEX_POINT ( 'NONE', #39490 ) ;
#30124=EDGE_LOOP ( 'NONE', ( #20018, #35060, #49750, #46740 ) ) ;
#30133=DIRECTION ( 'NONE',  ( -1.000000000000000000, 0.000000000000000000, -0.000000000000000000 ) ) ;
#30150=DIRECTION ( 'NONE',  ( 0.000000000000000000, 0.000000000000000000, -1.000000000000000000 ) ) ;
#30170=DIRECTION ( 'NONE',  ( -1.000000000000000000, 0.000000000000000000, 0.000000000000000000 ) ) ;
#30214=DIRECTION ( 'NONE',  ( 0.000000000000000000, -1.000000000000000000, 0.000000000000000000 ) ) ;
#30230=AXIS2_PLACEMENT_3D ( 'NONE', #36194, #32340, #40041 ) ;
#30232=LINE ( 'NONE', #33095, #50495 ) ;
#30234=ADVANCED_FACE ( 'NONE', ( #12517 ), #40235, .F. ) ;
#30278=EDGE_CURVE ( 'NONE', #9673, #4495, #28440, .T. ) ;
#30279=ORIENTED_EDGE ( 'NONE', *, *, #8769, .F. ) ;
#30310=ORIENTED_EDGE ( 'NONE', *, *, #10182, .F. ) ;
#30321=FACE_OUTER_BOUND ( 'NONE', #12860, .T. ) ;
#30323=EDGE_CURVE ( 'NONE', #9008, #5210, #45803, .T. ) ;
#30327=CARTESIAN_POINT ( 'NONE',  ( 177.5000000000000284, 112.5000000000000000, 0.000000000000000000 ) ) ;
#30432=CARTESIAN_POINT ( 'NONE',  ( -167.4999999999999432, -69.93075758371368522, -120.5992382549688671 ) ) ;
#30446=VECTOR ( 'NONE', #21476, 1000.000000000000000 ) ;
#30449=FACE_OUTER_BOUND ( 'NONE', #34107, .T. ) ;
#30457=PLANE ( 'NONE',  #48960 ) ;
#30463=DIRECTION ( 'NONE',  ( 0.000000000000000000, 0.000000000000000000, -1.000000000000000000 ) ) ;
#30472=CARTESIAN_POINT ( 'NONE',  ( -239.0000000000000853, -165.6999999999999602, 254.8599999999999852 ) ) ;
#30489=CARTESIAN_POINT ( 'NONE',  ( 214.9999999999999432, 173.0000000000000000, 112.0000000000000000 ) ) ;
#30501=EDGE_CURVE ( 'NONE', #15139, #11317, #50658, .T. ) ;
#30505=( BOUNDED_CURVE ( )  B_SPLINE_CURVE ( 3, ( #20091, #27556, #11380, #35780 ),
 .UNSPECIFIED., .F., .F. ) 
 B_SPLINE_CURVE_WITH_KNOTS ( ( 4, 4 ),
 ( 5.723266580096323608, 6.843104034262848856 ),
 .UNSPECIFIED. ) 
 CURVE ( )  GEOMETRIC_REPRESENTATION_ITEM ( )  RATIONAL_B_SPLINE_CURVE ( ( 1.000000000000000000, 0.8981988528445483677, 0.8981988528445483677, 1.000000000000000000 ) ) 
 REPRESENTATION_ITEM ( '' )  );
#30516=LINE ( 'NONE', #46884, #33930 ) ;
#30520=LINE ( 'NONE', #42560, #34717 ) ;
#30532=VERTEX_POINT ( 'NONE', #42243 ) ;
#30548=CIRCLE ( 'NONE', #37125, 40.00000000000000000 ) ;
#30551=CARTESIAN_POINT ( 'NONE',  ( 236.0000000000000000, -169.9999999999999716, 4.999999999999616307 ) ) ;
#30575=ADVANCED_FACE ( 'NONE', ( #30449 ), #46052, .F. ) ;
#30597=ORIENTED_EDGE ( 'NONE', *, *, #24146, .T. ) ;
#30618=PLANE ( 'NONE',  #28765 ) ;
#30651=CARTESIAN_POINT ( 'NONE',  ( 177.5000000000000284, -112.5000000000000000, -10.00000000000000000 ) ) ;
#30657=DIRECTION ( 'NONE',  ( -0.000000000000000000, -0.000000000000000000, -1.000000000000000000 ) ) ;
#30659=ADVANCED_FACE ( 'NONE', ( #39679 ), #47325, .F. ) ;
#30663=VECTOR ( 'NONE', #11047, 1000.000000000000000 ) ;
#30672=CARTESIAN_POINT ( 'NONE',  ( 194.9999999999999432, 173.0000000000000000, 132.0000000000000000 ) ) ;
#30754=CARTESIAN_POINT ( 'NONE',  ( -215.0000000000000568, 164.9999999999999716, 132.0000000000000000 ) ) ;
#30774=AXIS2_PLACEMENT_3D ( 'NONE', #50716, #4066, #15867 ) ;
#30814=ORIENTED_EDGE ( 'NONE', *, *, #41962, .T. ) ;
#30840=CARTESIAN_POINT ( 'NONE',  ( 0.000000000000000000, 175.0000000000000000, 500.0000000000001137 ) ) ;
#30878=VECTOR ( 'NONE', #16816, 1000.000000000000000 ) ;
#30917=CARTESIAN_POINT ( 'NONE',  ( -225.0000000000000568, -153.6999999999999602, 250.3600000000000136 ) ) ;
#30918=VECTOR ( 'NONE', #10438, 1000.000000000000000 ) ;
#30948=ORIENTED_EDGE ( 'NONE', *, *, #13368, .F. ) ;
#30957=ORIENTED_EDGE ( 'NONE', *, *, #45939, .F. ) ;
#30983=VERTEX_POINT ( 'NONE', #369 ) ;
#30994=CARTESIAN_POINT ( 'NONE',  ( 224.9999999999999716, -164.9999999999999716, 32.29650858650035161 ) ) ;
#31002=ORIENTED_EDGE ( 'NONE', *, *, #45602, .F. ) ;
#31005=EDGE_CURVE ( 'NONE', #48177, #32004, #41371, .T. ) ;
#31012=CARTESIAN_POINT ( 'NONE',  ( 194.9999999999999432, -173.0000000000000000, 112.0000000000000284 ) ) ;
#31021=CARTESIAN_POINT ( 'NONE',  ( -567.5000000000000000, -72.50000000000001421, -183.5999999999997954 ) ) ;
#31023=ORIENTED_EDGE ( 'NONE', *, *, #48140, .T. ) ;
#31036=DIRECTION ( 'NONE',  ( -1.000000000000000000, 0.000000000000000000, 0.000000000000000000 ) ) ;
#31040=ORIENTED_EDGE ( 'NONE', *, *, #37121, .T. ) ;
#31054=VERTEX_POINT ( 'NONE', #33188 ) ;
#31059=VERTEX_POINT ( 'NONE', #37047 ) ;
#31063=DIRECTION ( 'NONE',  ( 0.000000000000000000, 0.000000000000000000, -1.000000000000000000 ) ) ;
#31086=DIRECTION ( 'NONE',  ( -0.000000000000000000, -0.000000000000000000, 1.000000000000000000 ) ) ;
#31095=ORIENTED_EDGE ( 'NONE', *, *, #23748, .T. ) ;
#31126=FACE_OUTER_BOUND ( 'NONE', #14452, .T. ) ;
#31159=ADVANCED_FACE ( 'NONE', ( #24097 ), #244, .F. ) ;
#31181=ADVANCED_FACE ( 'NONE', ( #38304 ), #42112, .T. ) ;
#31183=CARTESIAN_POINT ( 'NONE',  ( 224.9999999999999432, 175.0000000000000000, 0.000000000000000000 ) ) ;
#31189=LINE ( 'NONE', #43725, #42262 ) ;
#31209=CARTESIAN_POINT ( 'NONE',  ( -215.0000000000000568, -175.0000000000000000, 500.0000000000000000 ) ) ;
#31216=EDGE_CURVE ( 'NONE', #11317, #22983, #47134, .T. ) ;
#31227=LINE ( 'NONE', #35090, #12608 ) ;
#31236=AXIS2_PLACEMENT_3D ( 'NONE', #36053, #34850, #23266 ) ;
#31238=CARTESIAN_POINT ( 'NONE',  ( -225.0000000000000568, 164.9999999999999716, 252.0000000000000000 ) ) ;
#31249=PLANE ( 'NONE',  #10903 ) ;
#31250=CARTESIAN_POINT ( 'NONE',  ( 0.000000000000000000, 0.000000000000000000, 910.0000000000000000 ) ) ;
#31251=VERTEX_POINT ( 'NONE', #10821 ) ;
#31270=CARTESIAN_POINT ( 'NONE',  ( -214.9999999999999432, 173.0000000000000000, 231.9999999999999716 ) ) ;
#31277=DIRECTION ( 'NONE',  ( 0.000000000000000000, -0.4436251537532894806, -0.8962124318248270161 ) ) ;
#31285=EDGE_CURVE ( 'NONE', #32625, #35472, #8701, .T. ) ;
#31303=AXIS2_PLACEMENT_3D ( 'NONE', #35971, #16457, #32108 ) ;
#31304=ADVANCED_FACE ( 'NONE', ( #48138 ), #17141, .F. ) ;
#31309=DIRECTION ( 'NONE',  ( 1.000000000000000000, 0.000000000000000000, 0.000000000000000000 ) ) ;
#31312=PLANE ( 'NONE',  #8989 ) ;
#31325=DIRECTION ( 'NONE',  ( -0.000000000000000000, -0.000000000000000000, 1.000000000000000000 ) ) ;
#31343=EDGE_CURVE ( 'NONE', #17183, #17041, #36153, .T. ) ;
#31354=CARTESIAN_POINT ( 'NONE',  ( -225.0000000000000568, -175.0000000000000000, 0.000000000000000000 ) ) ;
#31372=DIRECTION ( 'NONE',  ( 0.000000000000000000, -1.000000000000000000, 0.000000000000000000 ) ) ;
#31398=ORIENTED_EDGE ( 'NONE', *, *, #13313, .T. ) ;
#31445=VERTEX_POINT ( 'NONE', #38177 ) ;
#31462=LINE ( 'NONE', #27099, #33 ) ;
#31463=CARTESIAN_POINT ( 'NONE',  ( 232.4999999999999716, -169.9999999999999716, 444.9999999999998295 ) ) ;
#31466=ORIENTED_EDGE ( 'NONE', *, *, #5545, .F. ) ;
#31469=CARTESIAN_POINT ( 'NONE',  ( -239.0000000000000853, -153.6999999999999602, 250.3600000000000136 ) ) ;
#31475=AXIS2_PLACEMENT_3D ( 'NONE', #46664, #11563, #7717 ) ;
#31479=ADVANCED_FACE ( 'NONE', ( #37421 ), #17880, .F. ) ;
#31483=DIRECTION ( 'NONE',  ( -0.4055129968046615185, -0.4055129968046615185, -0.8192181753629524943 ) ) ;
#31503=ADVANCED_FACE ( 'NONE', ( #2740 ), #30457, .T. ) ;
#31515=EDGE_CURVE ( 'NONE', #18948, #40759, #26056, .T. ) ;
#31518=CARTESIAN_POINT ( 'NONE',  ( 0.000000000000000000, -50.00000000000000000, 900.0000000000000000 ) ) ;
#31519=ORIENTED_EDGE ( 'NONE', *, *, #40314, .F. ) ;
#31532=DIRECTION ( 'NONE',  ( 0.000000000000000000, -0.8962124318248270161, 0.4436251537532894806 ) ) ;
#31566=DIRECTION ( 'NONE',  ( 0.000000000000000000, 0.000000000000000000, 1.000000000000000000 ) ) ;
#31573=EDGE_LOOP ( 'NONE', ( #19268, #365, #48606, #19515 ) ) ;
#31606=EDGE_CURVE ( 'NONE', #25022, #2713, #27368, .T. ) ;
#31627=ORIENTED_EDGE ( 'NONE', *, *, #9042, .F. ) ;
#31637=AXIS2_PLACEMENT_3D ( 'NONE', #47350, #39207, #19936 ) ;
#31655=CARTESIAN_POINT ( 'NONE',  ( -33.89193117067290473, 21.24469349090191983, 910.0000000000000000 ) ) ;
#31657=VECTOR ( 'NONE', #44482, 1000.000000000000000 ) ;
#31679=PLANE ( 'NONE',  #41695 ) ;
#31688=EDGE_CURVE ( 'NONE', #10051, #26564, #21176, .T. ) ;
#31689=DIRECTION ( 'NONE',  ( 0.000000000000000000, -1.000000000000000000, -0.000000000000000000 ) ) ;
#31696=DIRECTION ( 'NONE',  ( -0.000000000000000000, -0.000000000000000000, 1.000000000000000000 ) ) ;
#31697=EDGE_LOOP ( 'NONE', ( #23204, #45902, #19634, #34049 ) ) ;
#31731=ORIENTED_EDGE ( 'NONE', *, *, #46857, .T. ) ;
#31740=EDGE_LOOP ( 'NONE', ( #16643, #20378, #44058, #43971 ) ) ;
#31741=PLANE ( 'NONE',  #29163 ) ;
#31758=DIRECTION ( 'NONE',  ( -1.000000000000000000, 0.000000000000000000, -0.000000000000000000 ) ) ;
#31770=ADVANCED_FACE ( 'NONE', ( #36353 ), #5018, .F. ) ;
#31771=CARTESIAN_POINT ( 'NONE',  ( -194.9999999999999432, 164.9999999999999716, 132.0000000000001137 ) ) ;
#31776=EDGE_LOOP ( 'NONE', ( #39963, #38269 ) ) ;
#31826=AXIS2_PLACEMENT_3D ( 'NONE', #42252, #3762, #4018 ) ;
#31886=LINE ( 'NONE', #4420, #9024 ) ;
#31923=CARTESIAN_POINT ( 'NONE',  ( 0.000000000000000000, 0.000000000000000000, 0.000000000000000000 ) ) ;
#31925=DIRECTION ( 'NONE',  ( 1.000000000000000000, 0.000000000000000000, 0.000000000000000000 ) ) ;
#31941=VECTOR ( 'NONE', #35639, 1000.000000000000000 ) ;
#31965=DIRECTION ( 'NONE',  ( -0.000000000000000000, -0.000000000000000000, -1.000000000000000000 ) ) ;
#31967=ORIENTED_EDGE ( 'NONE', *, *, #11541, .F. ) ;
#31975=CARTESIAN_POINT ( 'NONE',  ( -0.5000000000000000000, -0.5000000000000000000, 1000.000000000000000 ) ) ;
#31995=EDGE_CURVE ( 'NONE', #31059, #49554, #15264, .T. ) ;
#32004=VERTEX_POINT ( 'NONE', #4465 ) ;
#32023=DIRECTION ( 'NONE',  ( 0.000000000000000000, 0.000000000000000000, 1.000000000000000000 ) ) ;
#32080=VERTEX_POINT ( 'NONE', #378 ) ;
#32108=DIRECTION ( 'NONE',  ( -1.000000000000000000, 0.000000000000000000, 0.000000000000000000 ) ) ;
#32121=DIRECTION ( 'NONE',  ( 0.000000000000000000, -1.000000000000000000, 0.000000000000000000 ) ) ;
#32133=ORIENTED_EDGE ( 'NONE', *, *, #5778, .T. ) ;
#32145=LINE ( 'NONE', #47739, #23173 ) ;
#32157=DIRECTION ( 'NONE',  ( 0.1191452206184309831, 0.000000000000000000, -0.9928768384869219865 ) ) ;
#32161=ORIENTED_EDGE ( 'NONE', *, *, #37188, .F. ) ;
#32176=VERTEX_POINT ( 'NONE', #9814 ) ;
#32200=EDGE_CURVE ( 'NONE', #24673, #35472, #45694, .T. ) ;
#32210=ORIENTED_EDGE ( 'NONE', *, *, #39039, .T. ) ;
#32233=ADVANCED_FACE ( 'NONE', ( #5467, #33446 ), #2133, .F. ) ;
#32239=DIRECTION ( 'NONE',  ( 0.000000000000000000, 0.000000000000000000, 1.000000000000000000 ) ) ;
#32280=PLANE ( 'NONE',  #23506 ) ;
#32281=DIRECTION ( 'NONE',  ( 0.000000000000000000, 0.000000000000000000, 1.000000000000000000 ) ) ;
#32296=CARTESIAN_POINT ( 'NONE',  ( 432.7825420346616170, -102.8976013127941656, -7.208237214241163926 ) ) ;
#32301=CARTESIAN_POINT ( 'NONE',  ( 214.9999999999999432, 173.0000000000000000, 231.9999999999999716 ) ) ;
#32306=ORIENTED_EDGE ( 'NONE', *, *, #3020, .F. ) ;
#32309=CARTESIAN_POINT ( 'NONE',  ( 224.9999999999999432, -175.0000000000000000, 0.000000000000000000 ) ) ;
#32315=VECTOR ( 'NONE', #8222, 1000.000000000000000 ) ;
#32323=ORIENTED_EDGE ( 'NONE', *, *, #29958, .T. ) ;
#32324=VERTEX_POINT ( 'NONE', #34203 ) ;
#32340=DIRECTION ( 'NONE',  ( -0.000000000000000000, 0.000000000000000000, 1.000000000000000000 ) ) ;
#32382=CARTESIAN_POINT ( 'NONE',  ( 214.9999999999999432, -165.2931214222915628, 497.2965085865001811 ) ) ;
#32406=ORIENTED_EDGE ( 'NONE', *, *, #36825, .T. ) ;
#32409=LINE ( 'NONE', #12638, #40267 ) ;
#32418=ORIENTED_EDGE ( 'NONE', *, *, #13987, .F. ) ;
#32437=ADVANCED_FACE ( 'NONE', ( #1322 ), #43384, .T. ) ;
#32441=ORIENTED_EDGE ( 'NONE', *, *, #31515, .T. ) ;
#32443=EDGE_CURVE ( 'NONE', #37651, #49286, #12341, .T. ) ;
#32450=VECTOR ( 'NONE', #37347, 1000.000000000000000 ) ;
#32461=ORIENTED_EDGE ( 'NONE', *, *, #1747, .F. ) ;
#32514=ORIENTED_EDGE ( 'NONE', *, *, #32788, .T. ) ;
#32537=ORIENTED_EDGE ( 'NONE', *, *, #40330, .T. ) ;
#32549=CARTESIAN_POINT ( 'NONE',  ( 240.0000000000000000, -164.9999999999999716, 62.29650858650038003 ) ) ;
#32565=CARTESIAN_POINT ( 'NONE',  ( -37.90972275097262667, 14.83505920947805556, 901.8832493327278144 ) ) ;
#32581=ORIENTED_EDGE ( 'NONE', *, *, #30278, .F. ) ;
#32588=CARTESIAN_POINT ( 'NONE',  ( -33.89193117067293315, -33.89193117067293315, 910.0000000000000000 ) ) ;
#32594=LINE ( 'NONE', #48178, #39893 ) ;
#32603=CARTESIAN_POINT ( 'NONE',  ( 240.0000000000000000, -164.9999999999999716, 474.9999999999998863 ) ) ;
#32610=ORIENTED_EDGE ( 'NONE', *, *, #32954, .F. ) ;
#32625=VERTEX_POINT ( 'NONE', #22566 ) ;
#32648=ORIENTED_EDGE ( 'NONE', *, *, #26581, .F. ) ;
#32654=DIRECTION ( 'NONE',  ( -1.000000000000000000, 0.000000000000000000, 0.000000000000000000 ) ) ;
#32669=CARTESIAN_POINT ( 'NONE',  ( 224.9999999999999716, -164.9999999999999716, 62.29650858650038003 ) ) ;
#32713=LINE ( 'NONE', #9856, #32450 ) ;
#32724=AXIS2_PLACEMENT_3D ( 'NONE', #35602, #47590, #36102 ) ;
#32728=CARTESIAN_POINT ( 'NONE',  ( -194.9999999999999432, -173.0000000000000000, 132.0000000000000853 ) ) ;
#32731=ORIENTED_EDGE ( 'NONE', *, *, #34194, .F. ) ;
#32744=EDGE_CURVE ( 'NONE', #32625, #13604, #19985, .T. ) ;
#32788=EDGE_CURVE ( 'NONE', #32004, #14784, #28199, .T. ) ;
#32846=EDGE_CURVE ( 'NONE', #31251, #35508, #22444, .T. ) ;
#32854=ORIENTED_EDGE ( 'NONE', *, *, #29415, .T. ) ;
#32871=ORIENTED_EDGE ( 'NONE', *, *, #43711, .F. ) ;
#32874=DIRECTION ( 'NONE',  ( -1.000000000000000000, 0.000000000000000000, -0.000000000000000000 ) ) ;
#32892=LINE ( 'NONE', #5414, #10953 ) ;
#32896=CARTESIAN_POINT ( 'NONE',  ( 0.000000000000000000, 0.000000000000000000, 900.0000000000000000 ) ) ;
#32919=AXIS2_PLACEMENT_3D ( 'NONE', #25095, #48634, #33047 ) ;
#32921=CARTESIAN_POINT ( 'NONE',  ( 224.9999999999999716, -164.9999999999999716, 474.9999999999998863 ) ) ;
#32940=DIRECTION ( 'NONE',  ( 0.000000000000000000, 0.000000000000000000, -1.000000000000000000 ) ) ;
#32941=LINE ( 'NONE', #2128, #47084 ) ;
#32951=FACE_OUTER_BOUND ( 'NONE', #17452, .T. ) ;
#32954=EDGE_CURVE ( 'NONE', #49618, #30042, #33973, .T. ) ;
#32981=VECTOR ( 'NONE', #41738, 1000.000000000000000 ) ;
#32989=VECTOR ( 'NONE', #26809, 1000.000000000000000 ) ;
#33004=CARTESIAN_POINT ( 'NONE',  ( -225.0000000000000568, 164.9999999999999716, 132.0000000000000000 ) ) ;
#33012=LINE ( 'NONE', #48598, #4118 ) ;
#33029=CARTESIAN_POINT ( 'NONE',  ( -215.0000000000000568, 164.9999999999999716, 10.00000000000000000 ) ) ;
#33047=DIRECTION ( 'NONE',  ( 0.000000000000000000, 0.000000000000000000, 1.000000000000000000 ) ) ;
#33054=CARTESIAN_POINT ( 'NONE',  ( 0.000000000000000000, -164.9999999999999716, 0.000000000000000000 ) ) ;
#33060=VERTEX_POINT ( 'NONE', #46761 ) ;
#33095=CARTESIAN_POINT ( 'NONE',  ( 228.9999999999999716, -169.9999999999999716, 4.999999999999616307 ) ) ;
#33101=ADVANCED_FACE ( 'NONE', ( #24990, #32951 ), #1638, .T. ) ;
#33132=CIRCLE ( 'NONE', #44569, 50.00000000000000000 ) ;
#33143=PLANE ( 'NONE',  #13869 ) ;
#33176=CARTESIAN_POINT ( 'NONE',  ( -194.9999999999999432, 164.9999999999999716, 231.9999999999999147 ) ) ;
#33185=PLANE ( 'NONE',  #41391 ) ;
#33188=CARTESIAN_POINT ( 'NONE',  ( 236.0000000000000000, -169.9999999999999716, 444.9999999999998295 ) ) ;
#33189=LINE ( 'NONE', #44692, #28304 ) ;
#33250=CARTESIAN_POINT ( 'NONE',  ( 0.000000000000000000, 0.000000000000000000, 910.0000000000000000 ) ) ;
#33271=VECTOR ( 'NONE', #20032, 1000.000000000000000 ) ;
#33295=VERTEX_POINT ( 'NONE', #21627 ) ;
#33310=DIRECTION ( 'NONE',  ( 0.000000000000000000, 1.000000000000000000, -1.604368532695312981E-16 ) ) ;
#33332=ORIENTED_EDGE ( 'NONE', *, *, #27057, .T. ) ;
#33335=FACE_OUTER_BOUND ( 'NONE', #22842, .T. ) ;
#33369=ADVANCED_FACE ( 'NONE', ( #19029 ), #3898, .F. ) ;
#33409=EDGE_LOOP ( 'NONE', ( #28240, #1413, #34089, #27486 ) ) ;
#33446=FACE_BOUND ( 'NONE', #11640, .T. ) ;
#33455=CARTESIAN_POINT ( 'NONE',  ( 177.5000000000000284, -112.5000000000000000, -10.00000000000000000 ) ) ;
#33475=ORIENTED_EDGE ( 'NONE', *, *, #3828, .F. ) ;
#33485=EDGE_LOOP ( 'NONE', ( #47047, #5196, #35585, #49973 ) ) ;
#33490=ORIENTED_EDGE ( 'NONE', *, *, #2380, .F. ) ;
#33495=LINE ( 'NONE', #5774, #50655 ) ;
#33565=CARTESIAN_POINT ( 'NONE',  ( -0.5000000000000000000, 0.5000000000000000000, 1000.000000000000000 ) ) ;
#33573=DIRECTION ( 'NONE',  ( 0.000000000000000000, 1.000000000000000000, -1.604368532695312981E-16 ) ) ;
#33599=ORIENTED_EDGE ( 'NONE', *, *, #6428, .F. ) ;
#33608=CARTESIAN_POINT ( 'NONE',  ( 0.000000000000000000, -175.0000000000000000, 10.00000000000000000 ) ) ;
#33636=FACE_OUTER_BOUND ( 'NONE', #19954, .T. ) ;
#33652=VERTEX_POINT ( 'NONE', #3444 ) ;
#33672=EDGE_CURVE ( 'NONE', #48660, #12455, #26813, .T. ) ;
#33684=DIRECTION ( 'NONE',  ( -0.000000000000000000, -0.000000000000000000, -1.000000000000000000 ) ) ;
#33720=ORIENTED_EDGE ( 'NONE', *, *, #34901, .T. ) ;
#33734=EDGE_CURVE ( 'NONE', #13689, #43486, #15513, .T. ) ;
#33760=LINE ( 'NONE', #13227, #45788 ) ;
#33762=CARTESIAN_POINT ( 'NONE',  ( -167.4999999999999432, 47.50000000000000000, -10.00000000000000000 ) ) ;
#33776=DIRECTION ( 'NONE',  ( 0.000000000000000000, -1.000000000000000000, 1.604368532695312981E-16 ) ) ;
#33780=DIRECTION ( 'NONE',  ( 0.000000000000000000, 1.000000000000000000, 0.000000000000000000 ) ) ;
#33800=ORIENTED_EDGE ( 'NONE', *, *, #25789, .F. ) ;
#33810=LINE ( 'NONE', #14029, #8442 ) ;
#33821=CIRCLE ( 'NONE', #11687, 50.00000000000000000 ) ;
#33860=VECTOR ( 'NONE', #28994, 1000.000000000000000 ) ;
#33888=DIRECTION ( 'NONE',  ( 1.000000000000000000, 0.000000000000000000, -0.000000000000000000 ) ) ;
#33897=VECTOR ( 'NONE', #14748, 1000.000000000000000 ) ;
#33919=LINE ( 'NONE', #28361, #39415 ) ;
#33921=ORIENTED_EDGE ( 'NONE', *, *, #36825, .F. ) ;
#33930=VECTOR ( 'NONE', #11013, 1000.000000000000000 ) ;
#33931=DIRECTION ( 'NONE',  ( 0.000000000000000000, 1.000000000000000000, 0.000000000000000000 ) ) ;
#33940=CARTESIAN_POINT ( 'NONE',  ( -225.0000000000000568, -175.0000000000000000, 500.0000000000000000 ) ) ;
#33969=ORIENTED_EDGE ( 'NONE', *, *, #36185, .T. ) ;
#33973=( BOUNDED_CURVE ( )  B_SPLINE_CURVE ( 3, ( #26051, #32565, #1755, #28699 ),
 .UNSPECIFIED., .F., .F. ) 
 B_SPLINE_CURVE_WITH_KNOTS ( ( 4, 4 ),
 ( 5.723266580096323608, 6.283185307179586232 ),
 .UNSPECIFIED. ) 
 CURVE ( )  GEOMETRIC_REPRESENTATION_ITEM ( )  RATIONAL_B_SPLINE_CURVE ( ( 1.000000000000000000, 0.9740444450880465510, 0.9740444450880465510, 1.000000000000000000 ) ) 
 REPRESENTATION_ITEM ( '' )  );
#33979=EDGE_LOOP ( 'NONE', ( #3073, #14863, #24124, #27027 ) ) ;
#34001=CYLINDRICAL_SURFACE ( 'NONE', #12462, 3.500000000000003109 ) ;
#34029=VECTOR ( 'NONE', #622, 1000.000000000000000 ) ;
#34039=AXIS2_PLACEMENT_3D ( 'NONE', #8564, #366, #35522 ) ;
#34049=ORIENTED_EDGE ( 'NONE', *, *, #27702, .F. ) ;
#34060=ADVANCED_FACE ( 'NONE', ( #22142 ), #18529, .F. ) ;
#34069=DIRECTION ( 'NONE',  ( 0.000000000000000000, 1.000000000000000000, 0.000000000000000000 ) ) ;
#34087=CARTESIAN_POINT ( 'NONE',  ( 240.0000000000000000, -164.9999999999999716, 32.29650858650035161 ) ) ;
#34089=ORIENTED_EDGE ( 'NONE', *, *, #27707, .F. ) ;
#34097=LINE ( 'NONE', #45834, #5717 ) ;
#34099=AXIS2_PLACEMENT_3D ( 'NONE', #20392, #10110, #10374 ) ;
#34107=EDGE_LOOP ( 'NONE', ( #8274, #14039, #1366, #17341 ) ) ;
#34153=CARTESIAN_POINT ( 'NONE',  ( -225.0000000000000568, -165.6999999999999602, 250.3600000000000136 ) ) ;
#34188=CARTESIAN_POINT ( 'NONE',  ( 33.89193117067293315, -33.89193117067293315, 910.0000000000000000 ) ) ;
#34194=EDGE_CURVE ( 'NONE', #43155, #2713, #3900, .T. ) ;
#34196=CARTESIAN_POINT ( 'NONE',  ( 0.000000000000000000, 0.000000000000000000, 900.0000000000000000 ) ) ;
#34203=CARTESIAN_POINT ( 'NONE',  ( 33.89193117067290473, -21.24469349090191983, 910.0000000000000000 ) ) ;
#34265=CARTESIAN_POINT ( 'NONE',  ( 0.000000000000000000, 0.000000000000000000, 0.000000000000000000 ) ) ;
#34305=ADVANCED_FACE ( 'NONE', ( #1331 ), #1826, .T. ) ;
#34321=ORIENTED_EDGE ( 'NONE', *, *, #14208, .T. ) ;
#34352=LINE ( 'NONE', #14839, #12776 ) ;
#34358=ORIENTED_EDGE ( 'NONE', *, *, #26014, .F. ) ;
#34398=ORIENTED_EDGE ( 'NONE', *, *, #27365, .F. ) ;
#34411=ORIENTED_EDGE ( 'NONE', *, *, #32200, .T. ) ;
#34470=ORIENTED_EDGE ( 'NONE', *, *, #49656, .F. ) ;
#34482=ORIENTED_EDGE ( 'NONE', *, *, #50225, .T. ) ;
#34488=VECTOR ( 'NONE', #41714, 1000.000000000000114 ) ;
#34490=VECTOR ( 'NONE', #24242, 1000.000000000000000 ) ;
#34495=ORIENTED_EDGE ( 'NONE', *, *, #6325, .T. ) ;
#34500=ORIENTED_EDGE ( 'NONE', *, *, #23478, .F. ) ;
#34552=CARTESIAN_POINT ( 'NONE',  ( -177.4999999999999716, -112.5000000000000000, -10.00000000000000000 ) ) ;
#34555=CARTESIAN_POINT ( 'NONE',  ( 7.884183412771427868, 42.26678417219198991, 893.0811050474360400 ) ) ;
#34571=ORIENTED_EDGE ( 'NONE', *, *, #31995, .F. ) ;
#34575=CARTESIAN_POINT ( 'NONE',  ( 214.9999999999999432, -173.0000000000000000, 132.0000000000001137 ) ) ;
#34586=VERTEX_POINT ( 'NONE', #518 ) ;
#34598=DIRECTION ( 'NONE',  ( 0.000000000000000000, -1.000000000000000000, 8.021842663476564905E-17 ) ) ;
#34622=CARTESIAN_POINT ( 'NONE',  ( 224.9999999999999716, -164.9999999999999716, 32.29650858650035161 ) ) ;
#34630=CARTESIAN_POINT ( 'NONE',  ( 0.000000000000000000, 57.49999999999999289, 0.000000000000000000 ) ) ;
#34632=EDGE_CURVE ( 'NONE', #18292, #39878, #16647, .T. ) ;
#34636=FACE_OUTER_BOUND ( 'NONE', #26126, .T. ) ;
#34664=DIRECTION ( 'NONE',  ( -0.000000000000000000, -0.000000000000000000, 1.000000000000000000 ) ) ;
#34688=CARTESIAN_POINT ( 'NONE',  ( -215.0000000000000568, 164.9999999999999716, 231.9999999999999716 ) ) ;
#34691=FACE_OUTER_BOUND ( 'NONE', #23462, .T. ) ;
#34717=VECTOR ( 'NONE', #38495, 1000.000000000000000 ) ;
#34728=EDGE_CURVE ( 'NONE', #37995, #8296, #44829, .T. ) ;
#34729=CARTESIAN_POINT ( 'NONE',  ( -194.9999999999999432, 164.9999999999999716, 111.9999999999999858 ) ) ;
#34788=EDGE_CURVE ( 'NONE', #29488, #25367, #15339, .T. ) ;
#34803=LINE ( 'NONE', #27080, #29849 ) ;
#34805=ORIENTED_EDGE ( 'NONE', *, *, #34728, .F. ) ;
#34807=ORIENTED_EDGE ( 'NONE', *, *, #10461, .T. ) ;
#34821=FACE_OUTER_BOUND ( 'NONE', #27212, .T. ) ;
#34826=LINE ( 'NONE', #26085, #32981 ) ;
#34850=DIRECTION ( 'NONE',  ( -1.000000000000000000, 0.000000000000000000, 0.000000000000000000 ) ) ;
#34852=DIRECTION ( 'NONE',  ( -1.000000000000000000, 0.000000000000000000, 0.000000000000000000 ) ) ;
#34865=ADVANCED_FACE ( 'NONE', ( #50680 ), #20634, .T. ) ;
#34878=PLANE ( 'NONE',  #2866 ) ;
#34900=CARTESIAN_POINT ( 'NONE',  ( 214.9999999999999432, 164.9999999999999716, 497.2965085865001811 ) ) ;
#34901=EDGE_CURVE ( 'NONE', #21950, #3623, #19159, .T. ) ;
#34937=EDGE_CURVE ( 'NONE', #44965, #32324, #9590, .T. ) ;
#34940=DIRECTION ( 'NONE',  ( 0.000000000000000000, -1.000000000000000000, 1.604368532695312981E-16 ) ) ;
#34970=LINE ( 'NONE', #50535, #48457 ) ;
#34978=EDGE_LOOP ( 'NONE', ( #2065, #49469 ) ) ;
#34981=ORIENTED_EDGE ( 'NONE', *, *, #41736, .F. ) ;
#34985=ORIENTED_EDGE ( 'NONE', *, *, #45180, .T. ) ;
#35018=LINE ( 'NONE', #7804, #29598 ) ;
#35026=DIRECTION ( 'NONE',  ( 1.000000000000000000, 0.000000000000000000, 0.000000000000000000 ) ) ;
#35060=ORIENTED_EDGE ( 'NONE', *, *, #20555, .F. ) ;
#35065=EDGE_LOOP ( 'NONE', ( #22905, #39184, #8335, #28617 ) ) ;
#35078=DIRECTION ( 'NONE',  ( -1.000000000000000000, -0.000000000000000000, -0.000000000000000000 ) ) ;
#35082=ORIENTED_EDGE ( 'NONE', *, *, #37740, .F. ) ;
#35083=EDGE_LOOP ( 'NONE', ( #41205, #19749, #24136, #9265 ) ) ;
#35084=CARTESIAN_POINT ( 'NONE',  ( -21.24469349090191983, 33.89193117067290473, 910.0000000000000000 ) ) ;
#35085=DIRECTION ( 'NONE',  ( -0.000000000000000000, -0.000000000000000000, -1.000000000000000000 ) ) ;
#35090=CARTESIAN_POINT ( 'NONE',  ( -225.0000000000000568, -153.6999999999999602, 250.3600000000000136 ) ) ;
#35098=LINE ( 'NONE', #31238, #19275 ) ;
#35107=CARTESIAN_POINT ( 'NONE',  ( 224.9999999999999716, -164.9999999999999716, 32.29650858650035161 ) ) ;
#35108=LINE ( 'NONE', #11237, #11077 ) ;
#35140=CLOSED_SHELL ( 'NONE', ( #42473, #4755, #30659, #40083, #4478, #34305, #3230, #33369, #32233, #29417, #24396, #6713, #41240, #168, #34060, #14773, #18463, #29047, #32437, #24969, #44815, #5357, #17551, #9374, #31181, #47314, #35853, #4811, #28684, #8650, #6, #38169, #7179, #739, #42452, #35242, #36909, #26807, #20205, #1579, #41007, #35892, #34865, #17837, #2325, #8401, #6828, #18640, #509, #42544, #27443, #5636, #47777, #629, #8965, #4412, #24106, #16573, #2628, #3652, #1158, #42276, #30234, #9259, #38133, #31159, #24101, #31503, #33101, #27998, #47782, #16157, #17376, #41639, #6761, #31304, #30575, #31479, #45563, #17884, #7183, #48991, #9655, #8067, #31770, #11073, #20198, #41505, #10455, #24448, #50032, #41701, #48784, #14746, #16702, #22153, #15645, #37749, #14093, #13585, #3559, #42589, #14041, #893, #13897, #42792, #35579 ) ) ;
#35141=CARTESIAN_POINT ( 'NONE',  ( -177.4999999999999716, 74.83106485270648989, -130.5992382549688955 ) ) ;
#35150=EDGE_LOOP ( 'NONE', ( #45725, #18340, #10742, #39932, #2312, #31398 ) ) ;
#35181=CARTESIAN_POINT ( 'NONE',  ( -215.0000000000000568, -175.0000000000000000, 497.2965085865002379 ) ) ;
#35184=CARTESIAN_POINT ( 'NONE',  ( -225.0000000000000568, 164.9999999999999716, 231.9999999999999716 ) ) ;
#35202=CARTESIAN_POINT ( 'NONE',  ( -50.00000000000000000, 0.000000000000000000, 900.0000000000000000 ) ) ;
#35206=EDGE_LOOP ( 'NONE', ( #15490, #21268, #6364, #31002 ) ) ;
#35242=ADVANCED_FACE ( 'NONE', ( #27271 ), #3907, .T. ) ;
#35247=DIRECTION ( 'NONE',  ( 1.000000000000000000, 0.000000000000000000, 0.000000000000000000 ) ) ;
#35268=CARTESIAN_POINT ( 'NONE',  ( -177.4999999999999716, -112.5000000000000000, 0.000000000000000000 ) ) ;
#35277=EDGE_LOOP ( 'NONE', ( #48033, #39630, #43639, #42712 ) ) ;
#35326=VERTEX_POINT ( 'NONE', #25181 ) ;
#35330=CARTESIAN_POINT ( 'NONE',  ( 194.9999999999999432, 173.0000000000000000, 252.0000000000000000 ) ) ;
#35336=DIRECTION ( 'NONE',  ( 1.000000000000000000, 0.000000000000000000, 0.000000000000000000 ) ) ;
#35340=DIRECTION ( 'NONE',  ( 1.000000000000000000, 0.000000000000000000, 0.000000000000000000 ) ) ;
#35348=CARTESIAN_POINT ( 'NONE',  ( -325.0507910275983932, -325.0507910275983932, 321.8002831173224649 ) ) ;
#35357=CIRCLE ( 'NONE', #26319, 50.00000000000000000 ) ;
#35367=DIRECTION ( 'NONE',  ( 1.000000000000000000, 0.000000000000000000, 0.000000000000000000 ) ) ;
#35370=ORIENTED_EDGE ( 'NONE', *, *, #22353, .T. ) ;
#35388=VERTEX_POINT ( 'NONE', #29530 ) ;
#35421=VECTOR ( 'NONE', #40632, 1000.000000000000000 ) ;
#35427=VERTEX_POINT ( 'NONE', #45903 ) ;
#35429=ORIENTED_EDGE ( 'NONE', *, *, #26014, .T. ) ;
#35436=CARTESIAN_POINT ( 'NONE',  ( -50.00000000000000000, -50.00000000000000000, 900.0000000000000000 ) ) ;
#35446=AXIS2_PLACEMENT_3D ( 'NONE', #41615, #24970, #1619 ) ;
#35472=VERTEX_POINT ( 'NONE', #14893 ) ;
#35484=DIRECTION ( 'NONE',  ( 0.000000000000000000, -1.822804496942679766E-16, -1.000000000000000000 ) ) ;
#35490=DIRECTION ( 'NONE',  ( 0.000000000000000000, 0.9230769230769231282, 0.3846153846153844702 ) ) ;
#35506=LINE ( 'NONE', #27790, #7059 ) ;
#35508=VERTEX_POINT ( 'NONE', #14385 ) ;
#35522=DIRECTION ( 'NONE',  ( 0.000000000000000000, 0.000000000000000000, -1.000000000000000000 ) ) ;
#35550=ORIENTED_EDGE ( 'NONE', *, *, #44364, .F. ) ;
#35560=CARTESIAN_POINT ( 'NONE',  ( 224.9999999999999716, -175.0000000000000000, 444.9999999999998295 ) ) ;
#35567=CARTESIAN_POINT ( 'NONE',  ( 224.9999999999999432, -175.0000000000000000, 500.0000000000000000 ) ) ;
#35579=ADVANCED_FACE ( 'NONE', ( #3588 ), #38762, .T. ) ;
#35580=DIRECTION ( 'NONE',  ( 0.000000000000000000, -1.604368532695312981E-16, -1.000000000000000000 ) ) ;
#35585=ORIENTED_EDGE ( 'NONE', *, *, #1700, .T. ) ;
#35598=VECTOR ( 'NONE', #44520, 1000.000000000000000 ) ;
#35602=CARTESIAN_POINT ( 'NONE',  ( -194.9999999999999432, 173.0000000000000000, 231.9999999999999716 ) ) ;
#35607=ORIENTED_EDGE ( 'NONE', *, *, #18452, .F. ) ;
#35613=DIRECTION ( 'NONE',  ( 0.000000000000000000, 0.000000000000000000, -1.000000000000000000 ) ) ;
#35618=EDGE_LOOP ( 'NONE', ( #27583, #14246, #31519, #21018 ) ) ;
#35636=EDGE_LOOP ( 'NONE', ( #2463, #2830, #13849 ) ) ;
#35639=DIRECTION ( 'NONE',  ( 0.000000000000000000, -1.000000000000000000, 1.604368532695312981E-16 ) ) ;
#35654=VECTOR ( 'NONE', #26041, 1000.000000000000000 ) ;
#35662=DIRECTION ( 'NONE',  ( 0.000000000000000000, 0.000000000000000000, -1.000000000000000000 ) ) ;
#35698=ORIENTED_EDGE ( 'NONE', *, *, #27057, .F. ) ;
#35749=VECTOR ( 'NONE', #20129, 1000.000000000000000 ) ;
#35750=FACE_OUTER_BOUND ( 'NONE', #36110, .T. ) ;
#35780=CARTESIAN_POINT ( 'NONE',  ( 21.24469349090191983, -33.89193117067290473, 910.0000000000000000 ) ) ;
#35802=DIRECTION ( 'NONE',  ( 0.000000000000000000, -0.3846153846153845812, -0.9230769230769231282 ) ) ;
#35853=ADVANCED_FACE ( 'NONE', ( #41768 ), #41262, .F. ) ;
#35864=FACE_OUTER_BOUND ( 'NONE', #15888, .T. ) ;
#35871=ORIENTED_EDGE ( 'NONE', *, *, #43896, .T. ) ;
#35884=LINE ( 'NONE', #31270, #31941 ) ;
#35891=VERTEX_POINT ( 'NONE', #6622 ) ;
#35892=ADVANCED_FACE ( 'NONE', ( #33335 ), #6369, .T. ) ;
#35896=EDGE_CURVE ( 'NONE', #35472, #2521, #34097, .T. ) ;
#35916=EDGE_CURVE ( 'NONE', #10114, #6437, #22277, .T. ) ;
#35929=VECTOR ( 'NONE', #46184, 1000.000000000000000 ) ;
#35941=DIRECTION ( 'NONE',  ( -1.000000000000000000, 0.000000000000000000, 0.000000000000000000 ) ) ;
#35942=EDGE_CURVE ( 'NONE', #7894, #49308, #38452, .T. ) ;
#35963=DIRECTION ( 'NONE',  ( 0.000000000000000000, 0.000000000000000000, 1.000000000000000000 ) ) ;
#35971=CARTESIAN_POINT ( 'NONE',  ( 0.000000000000000000, 0.000000000000000000, 910.0000000000000000 ) ) ;
#35998=PLANE ( 'NONE',  #12724 ) ;
#36001=EDGE_LOOP ( 'NONE', ( #28786, #2482 ) ) ;
#36022=LINE ( 'NONE', #863, #6866 ) ;
#36027=VERTEX_POINT ( 'NONE', #39466 ) ;
#36032=CARTESIAN_POINT ( 'NONE',  ( 432.7825420346616170, -62.49999999999997158, -120.5992382549688671 ) ) ;
#36039=AXIS2_PLACEMENT_3D ( 'NONE', #22888, #14944, #19536 ) ;
#36051=VECTOR ( 'NONE', #18785, 1000.000000000000000 ) ;
#36053=CARTESIAN_POINT ( 'NONE',  ( 214.9999999999999432, -175.0000000000000000, 500.0000000000000000 ) ) ;
#36054=LINE ( 'NONE', #24494, #42568 ) ;
#36102=DIRECTION ( 'NONE',  ( 0.000000000000000000, 1.000000000000000000, -1.604368532695312981E-16 ) ) ;
#36110=EDGE_LOOP ( 'NONE', ( #34981, #37978, #21145 ) ) ;
#36119=ORIENTED_EDGE ( 'NONE', *, *, #42623, .T. ) ;
#36120=CARTESIAN_POINT ( 'NONE',  ( 240.0000000000000000, -164.9999999999999716, 474.9999999999998863 ) ) ;
#36122=ORIENTED_EDGE ( 'NONE', *, *, #19842, .T. ) ;
#36142=DIRECTION ( 'NONE',  ( 1.000000000000000000, 0.000000000000000000, 0.000000000000000000 ) ) ;
#36153=LINE ( 'NONE', #4818, #8054 ) ;
#36156=ORIENTED_EDGE ( 'NONE', *, *, #24112, .F. ) ;
#36182=FACE_OUTER_BOUND ( 'NONE', #39074, .T. ) ;
#36185=EDGE_CURVE ( 'NONE', #44566, #45963, #20703, .T. ) ;
#36194=CARTESIAN_POINT ( 'NONE',  ( 232.4999999999999716, -169.9999999999999716, 62.29650858650038003 ) ) ;
#36217=LINE ( 'NONE', #20043, #16323 ) ;
#36291=VECTOR ( 'NONE', #35336, 1000.000000000000000 ) ;
#36309=DIRECTION ( 'NONE',  ( 1.000000000000000000, -0.000000000000000000, -0.000000000000000000 ) ) ;
#36330=AXIS2_PLACEMENT_3D ( 'NONE', #7439, #11017, #3562 ) ;
#36338=ORIENTED_EDGE ( 'NONE', *, *, #16984, .F. ) ;
#36339=EDGE_CURVE ( 'NONE', #15139, #24711, #11187, .T. ) ;
#36353=FACE_OUTER_BOUND ( 'NONE', #7880, .T. ) ;
#36360=VECTOR ( 'NONE', #13984, 1000.000000000000000 ) ;
#36369=EDGE_LOOP ( 'NONE', ( #17213, #34482, #47877, #8117, #1297, #12914 ) ) ;
#36376=PLANE ( 'NONE',  #39407 ) ;
#36378=AXIS2_PLACEMENT_3D ( 'NONE', #35330, #35580, #3475 ) ;
#36419=DIRECTION ( 'NONE',  ( 0.9908916497796512735, 0.000000000000000000, 0.1346615698592613375 ) ) ;
#36425=CARTESIAN_POINT ( 'NONE',  ( 325.0507910275983932, -325.0507910275983932, 321.8002831173224649 ) ) ;
#36437=ORIENTED_EDGE ( 'NONE', *, *, #9943, .F. ) ;
#36453=VERTEX_POINT ( 'NONE', #28850 ) ;
#36495=ORIENTED_EDGE ( 'NONE', *, *, #40577, .F. ) ;
#36513=DIRECTION ( 'NONE',  ( 1.000000000000000000, 0.000000000000000000, 0.000000000000000000 ) ) ;
#36523=EDGE_CURVE ( 'NONE', #28864, #39878, #12190, .T. ) ;
#36527=ORIENTED_EDGE ( 'NONE', *, *, #300, .F. ) ;
#36531=FACE_OUTER_BOUND ( 'NONE', #29221, .T. ) ;
#36556=CARTESIAN_POINT ( 'NONE',  ( 224.9999999999999716, -164.9999999999999716, 62.29650858650038003 ) ) ;
#36566=VECTOR ( 'NONE', #49237, 1000.000000000000000 ) ;
#36623=CARTESIAN_POINT ( 'NONE',  ( 33.89193117067293315, 33.89193117067293315, 910.0000000000000000 ) ) ;
#36638=CYLINDRICAL_SURFACE ( 'NONE', #11024, 50.00000000000000000 ) ;
#36667=FACE_OUTER_BOUND ( 'NONE', #35150, .T. ) ;
#36668=CARTESIAN_POINT ( 'NONE',  ( 194.9999999999999716, 164.9999999999999716, 500.0000000000000000 ) ) ;
#36680=ORIENTED_EDGE ( 'NONE', *, *, #43353, .T. ) ;
#36681=DIRECTION ( 'NONE',  ( -0.000000000000000000, -0.000000000000000000, 1.000000000000000000 ) ) ;
#36701=EDGE_CURVE ( 'NONE', #44615, #48417, #27214, .T. ) ;
#36714=DIRECTION ( 'NONE',  ( -1.000000000000000000, -0.000000000000000000, -0.000000000000000000 ) ) ;
#36717=FACE_OUTER_BOUND ( 'NONE', #43188, .T. ) ;
#36729=DIRECTION ( 'NONE',  ( -1.000000000000000000, 0.000000000000000000, -0.000000000000000000 ) ) ;
#36761=EDGE_CURVE ( 'NONE', #32625, #1717, #15412, .T. ) ;
#36764=VERTEX_POINT ( 'NONE', #16417 ) ;
#36767=PLANE ( 'NONE',  #11161 ) ;
#36788=ORIENTED_EDGE ( 'NONE', *, *, #17913, .T. ) ;
#36817=DIRECTION ( 'NONE',  ( -0.000000000000000000, 1.000000000000000000, -1.604368532695312981E-16 ) ) ;
#36825=EDGE_CURVE ( 'NONE', #9839, #15483, #16939, .T. ) ;
#36849=VERTEX_POINT ( 'NONE', #1029 ) ;
#36852=VECTOR ( 'NONE', #23907, 1000.000000000000000 ) ;
#36869=CARTESIAN_POINT ( 'NONE',  ( 194.9999999999999432, -173.0000000000000000, 352.0000000000000568 ) ) ;
#36870=LINE ( 'NONE', #33004, #6098 ) ;
#36909=ADVANCED_FACE ( 'NONE', ( #48429 ), #9472, .T. ) ;
#36937=DIRECTION ( 'NONE',  ( -1.000000000000000000, 0.000000000000000000, 0.000000000000000000 ) ) ;
#36940=ORIENTED_EDGE ( 'NONE', *, *, #8693, .T. ) ;
#36964=VECTOR ( 'NONE', #24119, 1000.000000000000227 ) ;
#36965=ORIENTED_EDGE ( 'NONE', *, *, #31688, .T. ) ;
#36973=AXIS2_PLACEMENT_3D ( 'NONE', #9193, #28948, #9447 ) ;
#36991=DIRECTION ( 'NONE',  ( 0.000000000000000000, -1.000000000000000000, 0.000000000000000000 ) ) ;
#37006=DIRECTION ( 'NONE',  ( 0.000000000000000000, 0.000000000000000000, -1.000000000000000000 ) ) ;
#37047=CARTESIAN_POINT ( 'NONE',  ( -215.0000000000000568, 164.9999999999999716, 497.2965085865002379 ) ) ;
#37051=CARTESIAN_POINT ( 'NONE',  ( -225.0000000000000568, -175.0000000000000000, 0.000000000000000000 ) ) ;
#37104=DIRECTION ( 'NONE',  ( 0.000000000000000000, 0.2791762785758810650, -0.9602398687205827565 ) ) ;
#37109=FACE_OUTER_BOUND ( 'NONE', #20212, .T. ) ;
#37118=VECTOR ( 'NONE', #7475, 1000.000000000000000 ) ;
#37121=EDGE_CURVE ( 'NONE', #16638, #25367, #12162, .T. ) ;
#37124=DIRECTION ( 'NONE',  ( 0.9908916497796512735, -0.000000000000000000, 0.1346615698592613375 ) ) ;
#37125=AXIS2_PLACEMENT_3D ( 'NONE', #43895, #24423, #4405 ) ;
#37160=FACE_OUTER_BOUND ( 'NONE', #15307, .T. ) ;
#37172=DIRECTION ( 'NONE',  ( -1.000000000000000000, 0.000000000000000000, -0.000000000000000000 ) ) ;
#37180=LINE ( 'NONE', #25106, #4840 ) ;
#37188=EDGE_CURVE ( 'NONE', #1277, #32004, #13165, .T. ) ;
#37206=PLANE ( 'NONE',  #39855 ) ;
#37214=DIRECTION ( 'NONE',  ( 0.000000000000000000, 1.000000000000000000, -1.822804496942679766E-16 ) ) ;
#37231=ORIENTED_EDGE ( 'NONE', *, *, #12100, .T. ) ;
#37293=VERTEX_POINT ( 'NONE', #6981 ) ;
#37301=CARTESIAN_POINT ( 'NONE',  ( 194.9999999999999432, 173.0000000000000000, 112.0000000000000000 ) ) ;
#37324=EDGE_CURVE ( 'NONE', #45368, #39651, #22126, .T. ) ;
#37327=CARTESIAN_POINT ( 'NONE',  ( 177.5000000000000284, 102.5000000000000142, -8.474599139414886295 ) ) ;
#37341=DIRECTION ( 'NONE',  ( -0.000000000000000000, -1.000000000000000000, -0.000000000000000000 ) ) ;
#37347=DIRECTION ( 'NONE',  ( 0.000000000000000000, 1.000000000000000000, 0.000000000000000000 ) ) ;
#37356=PRODUCT_DEFINITION_FORMATION_WITH_SPECIFIED_SOURCE ( 'ANY', '', #44939, .NOT_KNOWN. ) ;
#37395=EDGE_LOOP ( 'NONE', ( #33599, #17351, #20189 ) ) ;
#37420=CARTESIAN_POINT ( 'NONE',  ( -239.0000000000000853, -165.6999999999999602, 254.8599999999999852 ) ) ;
#37421=FACE_OUTER_BOUND ( 'NONE', #47622, .T. ) ;
#37435=ORIENTED_EDGE ( 'NONE', *, *, #46995, .T. ) ;
#37451=FACE_OUTER_BOUND ( 'NONE', #46407, .T. ) ;
#37563=CARTESIAN_POINT ( 'NONE',  ( -225.0000000000000568, 175.0000000000000000, 500.0000000000000000 ) ) ;
#37606=DIRECTION ( 'NONE',  ( 0.000000000000000000, 0.2981428420003837121, 0.9545212652235329776 ) ) ;
#37610=DIRECTION ( 'NONE',  ( 1.000000000000000000, 0.000000000000000000, 0.000000000000000000 ) ) ;
#37612=CIRCLE ( 'NONE', #7298, 50.00000000000000000 ) ;
#37651=VERTEX_POINT ( 'NONE', #42060 ) ;
#37680=ORIENTED_EDGE ( 'NONE', *, *, #5614, .F. ) ;
#37692=DIRECTION ( 'NONE',  ( 0.000000000000000000, 0.000000000000000000, 1.000000000000000000 ) ) ;
#37696=DIRECTION ( 'NONE',  ( -0.000000000000000000, -0.000000000000000000, 1.000000000000000000 ) ) ;
#37740=EDGE_CURVE ( 'NONE', #41718, #16324, #30520, .T. ) ;
#37749=ADVANCED_FACE ( 'NONE', ( #34636 ), #18954, .T. ) ;
#37778=CARTESIAN_POINT ( 'NONE',  ( 194.9999999999999716, 164.9999999999999716, 132.0000000000001137 ) ) ;
#37843=DIRECTION ( 'NONE',  ( 1.000000000000000000, 0.000000000000000000, 0.000000000000000000 ) ) ;
#37844=ORIENTED_EDGE ( 'NONE', *, *, #40998, .F. ) ;
#37845=ORIENTED_EDGE ( 'NONE', *, *, #32788, .F. ) ;
#37849=DIRECTION ( 'NONE',  ( 0.000000000000000000, 1.000000000000000000, 0.000000000000000000 ) ) ;
#37963=DIRECTION ( 'NONE',  ( 1.000000000000000000, 0.000000000000000000, 0.000000000000000000 ) ) ;
#37978=ORIENTED_EDGE ( 'NONE', *, *, #4229, .T. ) ;
#37995=VERTEX_POINT ( 'NONE', #17835 ) ;
#38009=DIRECTION ( 'NONE',  ( 0.000000000000000000, -0.8962124318248270161, 0.4436251537532894806 ) ) ;
#38017=ORIENTED_EDGE ( 'NONE', *, *, #539, .F. ) ;
#38031=AXIS2_PLACEMENT_3D ( 'NONE', #5811, #48864, #21204 ) ;
#38034=VECTOR ( 'NONE', #37843, 1000.000000000000000 ) ;
#38044=DIRECTION ( 'NONE',  ( 0.1191452206184309970, 0.000000000000000000, -0.9928768384869220975 ) ) ;
#38076=EDGE_CURVE ( 'NONE', #9583, #15483, #46514, .T. ) ;
#38086=CARTESIAN_POINT ( 'NONE',  ( -50.00000000000000000, 50.00000000000000000, 900.0000000000000000 ) ) ;
#38098=FACE_OUTER_BOUND ( 'NONE', #13293, .T. ) ;
#38101=FACE_OUTER_BOUND ( 'NONE', #27248, .T. ) ;
#38106=CARTESIAN_POINT ( 'NONE',  ( 432.7825420346616170, 112.5000000000000000, -10.00000000000000178 ) ) ;
#38112=EDGE_CURVE ( 'NONE', #9583, #35891, #38877, .T. ) ;
#38120=CARTESIAN_POINT ( 'NONE',  ( 224.9999999999999716, -164.9999999999999716, 444.9999999999998295 ) ) ;
#38128=CARTESIAN_POINT ( 'NONE',  ( -177.4999999999999716, 112.5000000000000000, 0.000000000000000000 ) ) ;
#38133=ADVANCED_FACE ( 'NONE', ( #16271 ), #43461, .F. ) ;
#38164=DIRECTION ( 'NONE',  ( 0.000000000000000000, 1.000000000000000000, 0.000000000000000000 ) ) ;
#38169=ADVANCED_FACE ( 'NONE', ( #23719 ), #24233, .F. ) ;
#38177=CARTESIAN_POINT ( 'NONE',  ( -194.9999999999999432, -172.9999999999999716, 252.0000000000000568 ) ) ;
#38229=ORIENTED_EDGE ( 'NONE', *, *, #40577, .T. ) ;
#38267=AXIS2_PLACEMENT_3D ( 'NONE', #41269, #49684, #45838 ) ;
#38269=ORIENTED_EDGE ( 'NONE', *, *, #31515, .F. ) ;
#38272=ORIENTED_EDGE ( 'NONE', *, *, #1101, .T. ) ;
#38273=CARTESIAN_POINT ( 'NONE',  ( 194.9999999999999716, 164.9999999999999716, 500.0000000000000000 ) ) ;
#38294=LINE ( 'NONE', #6965, #12451 ) ;
#38304=FACE_OUTER_BOUND ( 'NONE', #777, .T. ) ;
#38305=CARTESIAN_POINT ( 'NONE',  ( -40.00000000000000000, 0.000000000000000000, 790.0000000000000000 ) ) ;
#38313=AXIS2_PLACEMENT_3D ( 'NONE', #32296, #28930, #40742 ) ;
#38338=ORIENTED_EDGE ( 'NONE', *, *, #36523, .T. ) ;
#38375=AXIS2_PLACEMENT_3D ( 'NONE', #34196, #35662, #15881 ) ;
#38376=FACE_OUTER_BOUND ( 'NONE', #8466, .T. ) ;
#38411=DIRECTION ( 'NONE',  ( 0.4740998230350172427, 0.3386427307392981256, -0.8127425537743157014 ) ) ;
#38430=DIRECTION ( 'NONE',  ( 0.000000000000000000, 0.000000000000000000, -1.000000000000000000 ) ) ;
#38452=LINE ( 'NONE', #46355, #18843 ) ;
#38488=( BOUNDED_CURVE ( )  B_SPLINE_CURVE ( 3, ( #1971, #17618, #48873, #13759 ),
 .UNSPECIFIED., .F., .F. ) 
 B_SPLINE_CURVE_WITH_KNOTS ( ( 4, 4 ),
 ( 0.000000000000000000, 0.5599187270832621799 ),
 .UNSPECIFIED. ) 
 CURVE ( )  GEOMETRIC_REPRESENTATION_ITEM ( )  RATIONAL_B_SPLINE_CURVE ( ( 1.000000000000000000, 0.9740444450880465510, 0.9740444450880465510, 1.000000000000000000 ) ) 
 REPRESENTATION_ITEM ( '' )  );
#38495=DIRECTION ( 'NONE',  ( 0.000000000000000000, -1.000000000000000000, 0.000000000000000000 ) ) ;
#38543=AXIS2_PLACEMENT_3D ( 'NONE', #13628, #38009, #2825 ) ;
#38572=VECTOR ( 'NONE', #23626, 1000.000000000000000 ) ;
#38607=DIRECTION ( 'NONE',  ( 0.000000000000000000, 1.000000000000000000, -1.604368532695312981E-16 ) ) ;
#38631=FACE_BOUND ( 'NONE', #39732, .T. ) ;
#38648=ORIENTED_EDGE ( 'NONE', *, *, #21120, .F. ) ;
#38650=ORIENTED_EDGE ( 'NONE', *, *, #49269, .F. ) ;
#38668=CARTESIAN_POINT ( 'NONE',  ( -215.0000000000000568, -165.7692307692307452, 496.1538461538461888 ) ) ;
#38683=VERTEX_POINT ( 'NONE', #34153 ) ;
#38684=LINE ( 'NONE', #18401, #11725 ) ;
#38690=FACE_OUTER_BOUND ( 'NONE', #23906, .T. ) ;
#38708=EDGE_CURVE ( 'NONE', #9008, #11165, #33821, .T. ) ;
#38711=CARTESIAN_POINT ( 'NONE',  ( 0.000000000000000000, -33.89193117067290473, 910.0000000000000000 ) ) ;
#38718=FACE_OUTER_BOUND ( 'NONE', #1223, .T. ) ;
#38762=PLANE ( 'NONE',  #49107 ) ;
#38819=DIRECTION ( 'NONE',  ( 0.000000000000000000, 0.000000000000000000, 1.000000000000000000 ) ) ;
#38826=FACE_OUTER_BOUND ( 'NONE', #18789, .T. ) ;
#38834=ORIENTED_EDGE ( 'NONE', *, *, #1747, .T. ) ;
#38858=EDGE_LOOP ( 'NONE', ( #46288, #7667, #47601, #26379, #43634, #998 ) ) ;
#38877=LINE ( 'NONE', #46261, #32989 ) ;
#38885=DIRECTION ( 'NONE',  ( 0.5038710255240862468, 0.000000000000000000, 0.8637789008984334549 ) ) ;
#38914=ORIENTED_EDGE ( 'NONE', *, *, #8874, .F. ) ;
#38921=AXIS2_PLACEMENT_3D ( 'NONE', #45802, #38164, #21984 ) ;
#38923=CARTESIAN_POINT ( 'NONE',  ( 21.24469349090191983, 33.89193117067290473, 910.0000000000000000 ) ) ;
#38942=CARTESIAN_POINT ( 'NONE',  ( 0.000000000000000000, 0.000000000000000000, 800.0000000000000000 ) ) ;
#38945=ORIENTED_EDGE ( 'NONE', *, *, #45696, .F. ) ;
#38968=CARTESIAN_POINT ( 'NONE',  ( -194.9999999999999432, 164.9999999999999716, 252.0000000000000000 ) ) ;
#38976=CARTESIAN_POINT ( 'NONE',  ( -21.24469349090191983, -33.89193117067290473, 910.0000000000000000 ) ) ;
#38977=ORIENTED_EDGE ( 'NONE', *, *, #1422, .T. ) ;
#38985=VECTOR ( 'NONE', #38411, 1000.000000000000000 ) ;
#38992=VERTEX_POINT ( 'NONE', #3002 ) ;
#39018=VECTOR ( 'NONE', #22532, 1000.000000000000000 ) ;
#39026=CARTESIAN_POINT ( 'NONE',  ( -177.4999999999999716, -77.43746236555679729, -130.5992382549688671 ) ) ;
#39038=ORIENTED_EDGE ( 'NONE', *, *, #17459, .T. ) ;
#39039=EDGE_CURVE ( 'NONE', #46103, #14468, #38684, .T. ) ;
#39046=EDGE_CURVE ( 'NONE', #44330, #20358, #49665, .T. ) ;
#39074=EDGE_LOOP ( 'NONE', ( #31466, #957, #48666, #33969 ) ) ;
#39085=DIRECTION ( 'NONE',  ( 0.000000000000000000, 0.000000000000000000, -1.000000000000000000 ) ) ;
#39099=CARTESIAN_POINT ( 'NONE',  ( -0.5000000000000000000, -0.5000000000000000000, 1000.000000000000000 ) ) ;
#39130=CARTESIAN_POINT ( 'NONE',  ( 0.000000000000000000, 0.000000000000000000, 800.0000000000000000 ) ) ;
#39144=ORIENTED_EDGE ( 'NONE', *, *, #14888, .F. ) ;
#39180=CARTESIAN_POINT ( 'NONE',  ( -167.4999999999999716, 74.83106485270648989, -120.5992382549688955 ) ) ;
#39184=ORIENTED_EDGE ( 'NONE', *, *, #5533, .T. ) ;
#39192=LINE ( 'NONE', #11225, #26157 ) ;
#39207=DIRECTION ( 'NONE',  ( 1.000000000000000000, 0.000000000000000000, 0.000000000000000000 ) ) ;
#39214=ORIENTED_EDGE ( 'NONE', *, *, #41354, .T. ) ;
#39217=CARTESIAN_POINT ( 'NONE',  ( 194.9999999999999716, 164.9999999999999716, 372.0000000000000000 ) ) ;
#39243=PLANE ( 'NONE',  #19148 ) ;
#39253=ORIENTED_EDGE ( 'NONE', *, *, #43353, .F. ) ;
#39258=VECTOR ( 'NONE', #6974, 1000.000000000000000 ) ;
#39267=EDGE_CURVE ( 'NONE', #39676, #19082, #45767, .T. ) ;
#39298=ORIENTED_EDGE ( 'NONE', *, *, #46995, .F. ) ;
#39308=EDGE_CURVE ( 'NONE', #1108, #47565, #18335, .T. ) ;
#39323=DIRECTION ( 'NONE',  ( 1.000000000000000000, 0.000000000000000000, -0.000000000000000000 ) ) ;
#39325=AXIS2_PLACEMENT_3D ( 'NONE', #22016, #10979, #21771 ) ;
#39337=FACE_OUTER_BOUND ( 'NONE', #35636, .T. ) ;
#39354=LINE ( 'NONE', #46996, #41131 ) ;
#39363=ORIENTED_EDGE ( 'NONE', *, *, #17673, .F. ) ;
#39371=( NAMED_UNIT ( * ) SI_UNIT ( $, .STERADIAN. ) SOLID_ANGLE_UNIT ( ) );
#39402=ORIENTED_EDGE ( 'NONE', *, *, #44948, .T. ) ;
#39407=AXIS2_PLACEMENT_3D ( 'NONE', #1216, #16862, #33776 ) ;
#39414=VERTEX_POINT ( 'NONE', #29783 ) ;
#39415=VECTOR ( 'NONE', #5255, 1000.000000000000000 ) ;
#39422=DIRECTION ( 'NONE',  ( 1.000000000000000000, 0.000000000000000000, 0.000000000000000000 ) ) ;
#39441=VECTOR ( 'NONE', #11899, 1000.000000000000000 ) ;
#39450=EDGE_CURVE ( 'NONE', #25022, #11648, #32892, .T. ) ;
#39466=CARTESIAN_POINT ( 'NONE',  ( 0.000000000000000000, 50.00000000000002132, 800.0000000000000000 ) ) ;
#39490=CARTESIAN_POINT ( 'NONE',  ( -225.0000000000000568, -153.6999999999999602, 254.8599999999999852 ) ) ;
#39491=CARTESIAN_POINT ( 'NONE',  ( -389.0218519071287346, 0.000000000000000000, 192.5658166940287970 ) ) ;
#39518=DIRECTION ( 'NONE',  ( -0.4740998230350174647, -0.3386427307392981256, -0.8127425537743155903 ) ) ;
#39554=ORIENTED_EDGE ( 'NONE', *, *, #39801, .F. ) ;
#39582=AXIS2_PLACEMENT_3D ( 'NONE', #41032, #5876, #37214 ) ;
#39591=EDGE_LOOP ( 'NONE', ( #26061, #45675, #12838, #11605, #16554 ) ) ;
#39593=ORIENTED_EDGE ( 'NONE', *, *, #44364, .T. ) ;
#39611=PRODUCT_DEFINITION_CONTEXT ( 'detailed design', #4994, 'design' ) ;
#39630=ORIENTED_EDGE ( 'NONE', *, *, #25021, .T. ) ;
#39633=ORIENTED_EDGE ( 'NONE', *, *, #31688, .F. ) ;
#39651=VERTEX_POINT ( 'NONE', #24373 ) ;
#39676=VERTEX_POINT ( 'NONE', #43093 ) ;
#39677=EDGE_CURVE ( 'NONE', #27283, #39414, #522, .T. ) ;
#39678=DIRECTION ( 'NONE',  ( 0.000000000000000000, -0.3846153846153845812, -0.9230769230769231282 ) ) ;
#39679=FACE_OUTER_BOUND ( 'NONE', #41573, .T. ) ;
#39694=DIRECTION ( 'NONE',  ( 0.000000000000000000, 0.000000000000000000, 1.000000000000000000 ) ) ;
#39697=DIRECTION ( 'NONE',  ( 0.000000000000000000, 0.000000000000000000, 1.000000000000000000 ) ) ;
#39724=PLANE ( 'NONE',  #47086 ) ;
#39725=LINE ( 'NONE', #4559, #29986 ) ;
#39732=EDGE_LOOP ( 'NONE', ( #25927, #33490, #10366, #23551 ) ) ;
#39768=DIRECTION ( 'NONE',  ( 0.000000000000000000, 0.000000000000000000, 1.000000000000000000 ) ) ;
#39769=LINE ( 'NONE', #16399, #7164 ) ;
#39801=EDGE_CURVE ( 'NONE', #35891, #31251, #9964, .T. ) ;
#39844=DIRECTION ( 'NONE',  ( 0.000000000000000000, 0.2981428420003837121, 0.9545212652235329776 ) ) ;
#39847=CARTESIAN_POINT ( 'NONE',  ( 0.5000000000000000000, 0.5000000000000000000, 1000.000000000000000 ) ) ;
#39855=AXIS2_PLACEMENT_3D ( 'NONE', #9467, #41028, #2710 ) ;
#39873=EDGE_LOOP ( 'NONE', ( #36122, #39905, #32648, #8171 ) ) ;
#39878=VERTEX_POINT ( 'NONE', #49424 ) ;
#39885=DIRECTION ( 'NONE',  ( -1.000000000000000000, 0.000000000000000000, 0.000000000000000000 ) ) ;
#39893=VECTOR ( 'NONE', #1787, 1000.000000000000000 ) ;
#39896=ORIENTED_EDGE ( 'NONE', *, *, #16285, .T. ) ;
#39904=ORIENTED_EDGE ( 'NONE', *, *, #22462, .T. ) ;
#39905=ORIENTED_EDGE ( 'NONE', *, *, #3691, .F. ) ;
#39906=CARTESIAN_POINT ( 'NONE',  ( -167.4999999999999432, 102.5000000000000142, -8.474599139414886295 ) ) ;
#39932=ORIENTED_EDGE ( 'NONE', *, *, #21751, .T. ) ;
#39941=CARTESIAN_POINT ( 'NONE',  ( -167.4999999999999432, 102.5000000000000142, -10.00000000000000000 ) ) ;
#39958=ORIENTED_EDGE ( 'NONE', *, *, #34788, .F. ) ;
#39963=ORIENTED_EDGE ( 'NONE', *, *, #3700, .F. ) ;
#39969=ORIENTED_EDGE ( 'NONE', *, *, #42623, .F. ) ;
#39996=VECTOR ( 'NONE', #18876, 1000.000000000000000 ) ;
#40002=DIRECTION ( 'NONE',  ( 0.000000000000000000, -0.000000000000000000, -1.000000000000000000 ) ) ;
#40008=LINE ( 'NONE', #48398, #43371 ) ;
#40022=ORIENTED_EDGE ( 'NONE', *, *, #13318, .F. ) ;
#40041=DIRECTION ( 'NONE',  ( 1.000000000000000000, 0.000000000000000000, 0.000000000000000000 ) ) ;
#40066=CARTESIAN_POINT ( 'NONE',  ( -214.9999999999999432, -173.0000000000000000, 112.0000000000000284 ) ) ;
#40083=ADVANCED_FACE ( 'NONE', ( #21196 ), #36638, .T. ) ;
#40084=LINE ( 'NONE', #43653, #4986 ) ;
#40087=DIRECTION ( 'NONE',  ( 0.4055129968046615185, 0.4055129968046615185, -0.8192181753629523833 ) ) ;
#40091=EDGE_CURVE ( 'NONE', #31059, #35508, #28902, .T. ) ;
#40099=LINE ( 'NONE', #17914, #8579 ) ;
#40110=CARTESIAN_POINT ( 'NONE',  ( 177.5000000000000284, -102.5000000000000142, 10.00000000000000000 ) ) ;
#40114=CARTESIAN_POINT ( 'NONE',  ( -225.0000000000000568, 164.9999999999999716, 352.0000000000000000 ) ) ;
#40115=DIRECTION ( 'NONE',  ( 1.000000000000000000, 0.000000000000000000, 0.000000000000000000 ) ) ;
#40142=EDGE_LOOP ( 'NONE', ( #39253, #27515, #16555, #11512, #22733, #21044, #1505, #50630, #32210, #36119 ) ) ;
#40146=ORIENTED_EDGE ( 'NONE', *, *, #16221, .F. ) ;
#40157=EDGE_CURVE ( 'NONE', #5061, #22675, #4879, .T. ) ;
#40235=PLANE ( 'NONE',  #38313 ) ;
#40267=VECTOR ( 'NONE', #28552, 1000.000000000000000 ) ;
#40284=ORIENTED_EDGE ( 'NONE', *, *, #22527, .F. ) ;
#40300=ORIENTED_EDGE ( 'NONE', *, *, #20169, .F. ) ;
#40307=EDGE_CURVE ( 'NONE', #9722, #28214, #1105, .T. ) ;
#40314=EDGE_CURVE ( 'NONE', #17183, #11317, #5946, .T. ) ;
#40330=EDGE_CURVE ( 'NONE', #44943, #11648, #5192, .T. ) ;
#40364=AXIS2_PLACEMENT_3D ( 'NONE', #50059, #2887, #7532 ) ;
#40399=DIRECTION ( 'NONE',  ( 0.000000000000000000, 1.000000000000000000, 0.000000000000000000 ) ) ;
#40404=CARTESIAN_POINT ( 'NONE',  ( -225.0000000000000568, -175.0000000000000000, 500.0000000000000000 ) ) ;
#40407=VERTEX_POINT ( 'NONE', #6963 ) ;
#40471=ORIENTED_EDGE ( 'NONE', *, *, #17706, .T. ) ;
#40514=VECTOR ( 'NONE', #327, 1000.000000000000000 ) ;
#40536=AXIS2_PLACEMENT_3D ( 'NONE', #26804, #49589, #42689 ) ;
#40537=ORIENTED_EDGE ( 'NONE', *, *, #12716, .T. ) ;
#40568=ORIENTED_EDGE ( 'NONE', *, *, #35942, .F. ) ;
#40577=EDGE_CURVE ( 'NONE', #28214, #30532, #4870, .T. ) ;
#40598=FACE_OUTER_BOUND ( 'NONE', #42223, .T. ) ;
#40613=DIRECTION ( 'NONE',  ( -1.000000000000000000, 0.000000000000000000, 0.000000000000000000 ) ) ;
#40616=VECTOR ( 'NONE', #30087, 1000.000000000000114 ) ;
#40628=LINE ( 'NONE', #43695, #47038 ) ;
#40632=DIRECTION ( 'NONE',  ( 0.000000000000000000, -1.000000000000000000, 0.000000000000000000 ) ) ;
#40674=ORIENTED_EDGE ( 'NONE', *, *, #13918, .F. ) ;
#40681=LINE ( 'NONE', #17571, #6732 ) ;
#40687=VECTOR ( 'NONE', #34940, 1000.000000000000000 ) ;
#40691=EDGE_LOOP ( 'NONE', ( #1404, #13964, #2357, #6320 ) ) ;
#40716=VECTOR ( 'NONE', #42533, 1000.000000000000000 ) ;
#40739=VECTOR ( 'NONE', #350, 1000.000000000000000 ) ;
#40742=DIRECTION ( 'NONE',  ( 0.000000000000000000, 0.2791762785758810650, -0.9602398687205827565 ) ) ;
#40745=DIRECTION ( 'NONE',  ( -0.000000000000000000, -0.000000000000000000, -1.000000000000000000 ) ) ;
#40759=VERTEX_POINT ( 'NONE', #10743 ) ;
#40763=CARTESIAN_POINT ( 'NONE',  ( -50.00000000000000000, -50.00000000000000000, 800.0000000000000000 ) ) ;
#40806=PLANE ( 'NONE',  #6180 ) ;
#40822=DIRECTION ( 'NONE',  ( -0.4055129968046615185, 0.4055129968046615185, -0.8192181753629524943 ) ) ;
#40831=VERTEX_POINT ( 'NONE', #18939 ) ;
#40836=DIRECTION ( 'NONE',  ( -0.000000000000000000, 1.604368532695312981E-16, 1.000000000000000000 ) ) ;
#40859=DIRECTION ( 'NONE',  ( 0.000000000000000000, -1.000000000000000000, 1.604368532695312981E-16 ) ) ;
#40862=EDGE_CURVE ( 'NONE', #11178, #2566, #15871, .T. ) ;
#40888=CARTESIAN_POINT ( 'NONE',  ( 33.89193117067290473, 0.000000000000000000, 910.0000000000000000 ) ) ;
#40894=AXIS2_PLACEMENT_3D ( 'NONE', #23119, #27237, #36729 ) ;
#40922=DIRECTION ( 'NONE',  ( 0.000000000000000000, 0.000000000000000000, 1.000000000000000000 ) ) ;
#40956=ORIENTED_EDGE ( 'NONE', *, *, #30323, .T. ) ;
#40958=ORIENTED_EDGE ( 'NONE', *, *, #31005, .T. ) ;
#40975=ORIENTED_EDGE ( 'NONE', *, *, #17673, .T. ) ;
#40998=EDGE_CURVE ( 'NONE', #39878, #35427, #20463, .T. ) ;
#41002=DIRECTION ( 'NONE',  ( 0.000000000000000000, -1.000000000000000000, 0.000000000000000000 ) ) ;
#41007=ADVANCED_FACE ( 'NONE', ( #37160 ), #49879, .F. ) ;
#41023=ORIENTED_EDGE ( 'NONE', *, *, #2486, .T. ) ;
#41028=DIRECTION ( 'NONE',  ( 1.000000000000000000, 0.000000000000000000, -0.000000000000000000 ) ) ;
#41029=LINE ( 'NONE', #17424, #28206 ) ;
#41032=CARTESIAN_POINT ( 'NONE',  ( 432.7825420346616170, 74.83106485270648989, -130.5992382549688955 ) ) ;
#41043=AXIS2_PLACEMENT_3D ( 'NONE', #18332, #30150, #25546 ) ;
#41078=VECTOR ( 'NONE', #10457, 1000.000000000000000 ) ;
#41092=DIRECTION ( 'NONE',  ( 0.000000000000000000, 0.000000000000000000, 1.000000000000000000 ) ) ;
#41131=VECTOR ( 'NONE', #356, 1000.000000000000000 ) ;
#41155=CARTESIAN_POINT ( 'NONE',  ( -50.00000000000000000, -50.00000000000000000, 800.0000000000000000 ) ) ;
#41159=VECTOR ( 'NONE', #42105, 1000.000000000000000 ) ;
#41171=VECTOR ( 'NONE', #16549, 1000.000000000000000 ) ;
#41205=ORIENTED_EDGE ( 'NONE', *, *, #29958, .F. ) ;
#41238=EDGE_CURVE ( 'NONE', #1180, #44943, #20324, .T. ) ;
#41240=ADVANCED_FACE ( 'NONE', ( #15556 ), #11703, .F. ) ;
#41257=ORIENTED_EDGE ( 'NONE', *, *, #14651, .T. ) ;
#41260=VERTEX_POINT ( 'NONE', #1432 ) ;
#41262=PLANE ( 'NONE',  #39325 ) ;
#41269=CARTESIAN_POINT ( 'NONE',  ( 194.9999999999999432, 173.0000000000000000, 372.0000000000000000 ) ) ;
#41296=VECTOR ( 'NONE', #40745, 1000.000000000000000 ) ;
#41299=CARTESIAN_POINT ( 'NONE',  ( 0.000000000000000000, 43.33333333333339255, 790.0000000000000000 ) ) ;
#41306=CARTESIAN_POINT ( 'NONE',  ( 0.000000000000000000, 164.9999999999999716, 10.00000000000000000 ) ) ;
#41337=CARTESIAN_POINT ( 'NONE',  ( 0.000000000000000000, 0.000000000000000000, 790.0000000000000000 ) ) ;
#41354=EDGE_CURVE ( 'NONE', #30042, #17677, #1677, .T. ) ;
#41371=LINE ( 'NONE', #1874, #24460 ) ;
#41390=CARTESIAN_POINT ( 'NONE',  ( -239.0000000000000853, -165.6999999999999602, 250.3600000000000136 ) ) ;
#41391=AXIS2_PLACEMENT_3D ( 'NONE', #37301, #18946, #45179 ) ;
#41433=LINE ( 'NONE', #6295, #10200 ) ;
#41434=EDGE_LOOP ( 'NONE', ( #43983, #4244 ) ) ;
#41474=CIRCLE ( 'NONE', #26755, 50.00000000000000000 ) ;
#41476=CARTESIAN_POINT ( 'NONE',  ( 0.000000000000000000, 389.0218519071287346, 192.5658166940287970 ) ) ;
#41478=AXIS2_PLACEMENT_3D ( 'NONE', #31463, #7351, #49874 ) ;
#41505=ADVANCED_FACE ( 'NONE', ( #18566 ), #11649, .F. ) ;
#41518=EDGE_CURVE ( 'NONE', #36849, #7843, #15742, .T. ) ;
#41573=EDGE_LOOP ( 'NONE', ( #25643, #24548, #11557, #48949, #45986, #721, #43394, #25630 ) ) ;
#41595=ORIENTED_EDGE ( 'NONE', *, *, #16221, .T. ) ;
#41615=CARTESIAN_POINT ( 'NONE',  ( 0.000000000000000000, -326.6272189349111841, 136.0946745562129649 ) ) ;
#41639=ADVANCED_FACE ( 'NONE', ( #4453 ), #16758, .T. ) ;
#41655=VECTOR ( 'NONE', #31483, 1000.000000000000114 ) ;
#41668=ORIENTED_EDGE ( 'NONE', *, *, #39677, .F. ) ;
#41673=CARTESIAN_POINT ( 'NONE',  ( 50.00000000000000000, -50.00000000000000000, 900.0000000000000000 ) ) ;
#41674=ORIENTED_EDGE ( 'NONE', *, *, #25844, .T. ) ;
#41689=VECTOR ( 'NONE', #12535, 1000.000000000000000 ) ;
#41695=AXIS2_PLACEMENT_3D ( 'NONE', #7288, #7552, #50598 ) ;
#41699=FACE_OUTER_BOUND ( 'NONE', #37395, .T. ) ;
#41701=ADVANCED_FACE ( 'NONE', ( #15115 ), #33185, .F. ) ;
#41714=DIRECTION ( 'NONE',  ( -0.9928768384869219865, 0.000000000000000000, -0.1191452206184307611 ) ) ;
#41718=VERTEX_POINT ( 'NONE', #25981 ) ;
#41736=EDGE_CURVE ( 'NONE', #16113, #11215, #14149, .T. ) ;
#41738=DIRECTION ( 'NONE',  ( 0.000000000000000000, 1.000000000000000000, 0.000000000000000000 ) ) ;
#41750=CARTESIAN_POINT ( 'NONE',  ( 167.5000000000000000, -112.5000000000000000, 10.00000000000000000 ) ) ;
#41760=EDGE_CURVE ( 'NONE', #43789, #48660, #49267, .T. ) ;
#41762=CARTESIAN_POINT ( 'NONE',  ( 194.9999999999999432, 173.0000000000000000, 352.0000000000000000 ) ) ;
#41768=FACE_OUTER_BOUND ( 'NONE', #5641, .T. ) ;
#41783=ORIENTED_EDGE ( 'NONE', *, *, #10182, .T. ) ;
#41792=CARTESIAN_POINT ( 'NONE',  ( -582.5000000000000000, 47.50000000000000000, -58.60000000000003695 ) ) ;
#41802=AXIS2_PLACEMENT_3D ( 'NONE', #27232, #6964, #23375 ) ;
#41821=ORIENTED_EDGE ( 'NONE', *, *, #4563, .F. ) ;
#41841=LINE ( 'NONE', #2828, #30663 ) ;
#41854=ORIENTED_EDGE ( 'NONE', *, *, #16741, .T. ) ;
#41892=ORIENTED_EDGE ( 'NONE', *, *, #20555, .T. ) ;
#41907=VERTEX_POINT ( 'NONE', #19463 ) ;
#41953=DIRECTION ( 'NONE',  ( -1.000000000000000000, 0.000000000000000000, 0.000000000000000000 ) ) ;
#41954=FACE_OUTER_BOUND ( 'NONE', #47907, .T. ) ;
#41957=LINE ( 'NONE', #3968, #43006 ) ;
#41962=EDGE_CURVE ( 'NONE', #1551, #20787, #47636, .T. ) ;
#42006=CARTESIAN_POINT ( 'NONE',  ( 232.4999999999999716, -169.9999999999999716, 444.9999999999998295 ) ) ;
#42016=CARTESIAN_POINT ( 'NONE',  ( 177.5000000000000284, 102.5000000000000142, 10.00000000000000000 ) ) ;
#42018=ORIENTED_EDGE ( 'NONE', *, *, #17139, .T. ) ;
#42060=CARTESIAN_POINT ( 'NONE',  ( 224.9999999999999716, -164.9999999999999716, 444.9999999999998295 ) ) ;
#42074=VERTEX_POINT ( 'NONE', #6090 ) ;
#42079=CARTESIAN_POINT ( 'NONE',  ( -581.3085477938157055, -62.49999999999998579, -68.52876838486925237 ) ) ;
#42091=DIRECTION ( 'NONE',  ( -1.000000000000000000, 0.000000000000000000, 0.000000000000000000 ) ) ;
#42097=PLANE ( 'NONE',  #41802 ) ;
#42105=DIRECTION ( 'NONE',  ( -1.000000000000000000, -0.000000000000000000, 0.000000000000000000 ) ) ;
#42112=PLANE ( 'NONE',  #38375 ) ;
#42118=LINE ( 'NONE', #26482, #14917 ) ;
#42147=VECTOR ( 'NONE', #29053, 1000.000000000000000 ) ;
#42217=CARTESIAN_POINT ( 'NONE',  ( -194.9999999999999432, 173.0000000000000000, 112.0000000000000000 ) ) ;
#42223=EDGE_LOOP ( 'NONE', ( #8036, #47876, #34805, #48226 ) ) ;
#42227=LINE ( 'NONE', #15032, #48693 ) ;
#42243=CARTESIAN_POINT ( 'NONE',  ( 224.9999999999999716, -175.0000000000000000, 474.9999999999998863 ) ) ;
#42247=ORIENTED_EDGE ( 'NONE', *, *, #35896, .F. ) ;
#42252=CARTESIAN_POINT ( 'NONE',  ( 232.4999999999999716, -169.9999999999999716, 62.29650858650038003 ) ) ;
#42262=VECTOR ( 'NONE', #15284, 1000.000000000000000 ) ;
#42276=ADVANCED_FACE ( 'NONE', ( #11977 ), #31741, .F. ) ;
#42295=ORIENTED_EDGE ( 'NONE', *, *, #12252, .F. ) ;
#42339=CARTESIAN_POINT ( 'NONE',  ( 236.0000000000000000, -169.9999999999999716, 4.999999999999616307 ) ) ;
#42380=DIRECTION ( 'NONE',  ( 0.000000000000000000, 1.000000000000000000, 0.000000000000000000 ) ) ;
#42393=VERTEX_POINT ( 'NONE', #24531 ) ;
#42445=VERTEX_POINT ( 'NONE', #48836 ) ;
#42449=DIRECTION ( 'NONE',  ( -1.000000000000000000, 0.000000000000000000, -0.000000000000000000 ) ) ;
#42452=ADVANCED_FACE ( 'NONE', ( #13726 ), #45251, .T. ) ;
#42473=ADVANCED_FACE ( 'NONE', ( #37109 ), #34001, .F. ) ;
#42533=DIRECTION ( 'NONE',  ( 0.000000000000000000, -1.000000000000000000, 1.822804496942679766E-16 ) ) ;
#42537=EDGE_LOOP ( 'NONE', ( #26259, #38650, #5677, #38272 ) ) ;
#42544=ADVANCED_FACE ( 'NONE', ( #3433 ), #19598, .F. ) ;
#42555=VECTOR ( 'NONE', #37006, 1000.000000000000000 ) ;
#42557=CARTESIAN_POINT ( 'NONE',  ( 194.9999999999999432, -173.0000000000000000, 112.0000000000000284 ) ) ;
#42560=CARTESIAN_POINT ( 'NONE',  ( -167.4999999999999432, -112.5000000000000000, -18.87174264961130632 ) ) ;
#42565=EDGE_CURVE ( 'NONE', #36027, #16851, #5902, .T. ) ;
#42568=VECTOR ( 'NONE', #36309, 1000.000000000000000 ) ;
#42589=ADVANCED_FACE ( 'NONE', ( #43208 ), #23715, .T. ) ;
#42623=EDGE_CURVE ( 'NONE', #14468, #9223, #28319, .T. ) ;
#42644=ORIENTED_EDGE ( 'NONE', *, *, #40157, .F. ) ;
#42658=PLANE ( 'NONE',  #40364 ) ;
#42666=AXIS2_PLACEMENT_3D ( 'NONE', #11871, #20067, #12127 ) ;
#42689=DIRECTION ( 'NONE',  ( -1.000000000000000000, 0.000000000000000000, 0.000000000000000000 ) ) ;
#42701=ORIENTED_EDGE ( 'NONE', *, *, #13283, .F. ) ;
#42712=ORIENTED_EDGE ( 'NONE', *, *, #5109, .F. ) ;
#42720=ORIENTED_EDGE ( 'NONE', *, *, #453, .F. ) ;
#42755=DIRECTION ( 'NONE',  ( -1.000000000000000000, 0.000000000000000000, -0.000000000000000000 ) ) ;
#42785=ORIENTED_EDGE ( 'NONE', *, *, #35916, .F. ) ;
#42792=ADVANCED_FACE ( 'NONE', ( #48523 ), #5714, .T. ) ;
#42810=FACE_OUTER_BOUND ( 'NONE', #45932, .T. ) ;
#42811=VECTOR ( 'NONE', #38044, 999.9999999999998863 ) ;
#42858=FACE_OUTER_BOUND ( 'NONE', #31697, .T. ) ;
#42892=VECTOR ( 'NONE', #16817, 1000.000000000000000 ) ;
#42900=UNCERTAINTY_MEASURE_WITH_UNIT (LENGTH_MEASURE( 1.000000000000000082E-05 ), #50597, 'distance_accuracy_value', 'NONE');
#42903=EDGE_CURVE ( 'NONE', #6362, #13604, #42118, .T. ) ;
#42914=LINE ( 'NONE', #47245, #22700 ) ;
#42928=ORIENTED_EDGE ( 'NONE', *, *, #49840, .T. ) ;
#42944=CARTESIAN_POINT ( 'NONE',  ( 167.5000000000000000, -69.93075758371368522, -120.5992382549688671 ) ) ;
#42945=EDGE_CURVE ( 'NONE', #11648, #49618, #34970, .T. ) ;
#42966=ORIENTED_EDGE ( 'NONE', *, *, #20417, .F. ) ;
#42971=ORIENTED_EDGE ( 'NONE', *, *, #16285, .F. ) ;
#42993=DIRECTION ( 'NONE',  ( 0.000000000000000000, 0.000000000000000000, -1.000000000000000000 ) ) ;
#43006=VECTOR ( 'NONE', #45772, 1000.000000000000000 ) ;
#43015=CARTESIAN_POINT ( 'NONE',  ( 240.0000000000000000, -175.0000000000000000, 32.29650858650035161 ) ) ;
#43019=FACE_OUTER_BOUND ( 'NONE', #29239, .T. ) ;
#43025=VECTOR ( 'NONE', #3164, 1000.000000000000000 ) ;
#43026=PLANE ( 'NONE',  #31637 ) ;
#43049=LINE ( 'NONE', #7418, #2901 ) ;
#43055=VECTOR ( 'NONE', #19522, 1000.000000000000000 ) ;
#43093=CARTESIAN_POINT ( 'NONE',  ( 214.9999999999999432, 164.9999999999999716, 111.9999999999999858 ) ) ;
#43129=EDGE_CURVE ( 'NONE', #40831, #17041, #8253, .T. ) ;
#43131=VECTOR ( 'NONE', #13388, 1000.000000000000000 ) ;
#43134=ORIENTED_EDGE ( 'NONE', *, *, #6765, .F. ) ;
#43137=CARTESIAN_POINT ( 'NONE',  ( 21.24469349090191983, 33.89193117067290473, 910.0000000000000000 ) ) ;
#43141=EDGE_CURVE ( 'NONE', #33295, #32324, #43544, .T. ) ;
#43155=VERTEX_POINT ( 'NONE', #29260 ) ;
#43164=PLANE ( 'NONE',  #49050 ) ;
#43188=EDGE_LOOP ( 'NONE', ( #50686, #39402, #9602, #20876, #47661 ) ) ;
#43195=EDGE_LOOP ( 'NONE', ( #35429, #6267, #21070 ) ) ;
#43200=FACE_OUTER_BOUND ( 'NONE', #35083, .T. ) ;
#43208=FACE_OUTER_BOUND ( 'NONE', #19385, .T. ) ;
#43254=LINE ( 'NONE', #3753, #23069 ) ;
#43261=CARTESIAN_POINT ( 'NONE',  ( 331.7552636306688214, -248.6897383013408103, 297.1446280767819985 ) ) ;
#43285=CARTESIAN_POINT ( 'NONE',  ( 167.5000000000000000, -102.5000000000000142, 10.00000000000000000 ) ) ;
#43302=LINE ( 'NONE', #31021, #22141 ) ;
#43310=FACE_OUTER_BOUND ( 'NONE', #49856, .T. ) ;
#43331=LINE ( 'NONE', #27448, #15542 ) ;
#43353=EDGE_CURVE ( 'NONE', #11178, #9223, #11019, .T. ) ;
#43354=VERTEX_POINT ( 'NONE', #34900 ) ;
#43371=VECTOR ( 'NONE', #36419, 1000.000000000000114 ) ;
#43384=PLANE ( 'NONE',  #11402 ) ;
#43394=ORIENTED_EDGE ( 'NONE', *, *, #16222, .T. ) ;
#43414=LINE ( 'NONE', #11360, #20180 ) ;
#43420=CARTESIAN_POINT ( 'NONE',  ( -214.5896300087917155, 164.9999999999999716, 498.0000000000002274 ) ) ;
#43429=DIRECTION ( 'NONE',  ( 0.000000000000000000, -1.000000000000000000, 0.000000000000000000 ) ) ;
#43461=PLANE ( 'NONE',  #2630 ) ;
#43486=VERTEX_POINT ( 'NONE', #45045 ) ;
#43507=CARTESIAN_POINT ( 'NONE',  ( 0.000000000000000000, 0.000000000000000000, 900.0000000000000000 ) ) ;
#43544=CIRCLE ( 'NONE', #31303, 40.00000000000000000 ) ;
#43555=DIRECTION ( 'NONE',  ( 1.000000000000000000, 0.000000000000000000, 0.000000000000000000 ) ) ;
#43566=DIRECTION ( 'NONE',  ( 0.000000000000000000, 0.000000000000000000, -1.000000000000000000 ) ) ;
#43589=AXIS2_PLACEMENT_3D ( 'NONE', #23464, #30657, #47016 ) ;
#43607=CARTESIAN_POINT ( 'NONE',  ( -581.3085477938158192, 57.49999999999996447, -68.52876838486925237 ) ) ;
#43634=ORIENTED_EDGE ( 'NONE', *, *, #21751, .F. ) ;
#43636=DIRECTION ( 'NONE',  ( 1.000000000000000000, 0.000000000000000000, 0.000000000000000000 ) ) ;
#43639=ORIENTED_EDGE ( 'NONE', *, *, #39046, .F. ) ;
#43641=ORIENTED_EDGE ( 'NONE', *, *, #20169, .T. ) ;
#43652=VECTOR ( 'NONE', #5967, 1000.000000000000000 ) ;
#43653=CARTESIAN_POINT ( 'NONE',  ( 177.5000000000000000, 112.5000000000000000, -10.00000000000000178 ) ) ;
#43678=VECTOR ( 'NONE', #22436, 1000.000000000000000 ) ;
#43695=CARTESIAN_POINT ( 'NONE',  ( 0.000000000000000000, -33.89193117067290473, 910.0000000000000000 ) ) ;
#43704=EDGE_CURVE ( 'NONE', #15488, #37293, #97, .T. ) ;
#43711=EDGE_CURVE ( 'NONE', #4061, #45368, #39354, .T. ) ;
#43725=CARTESIAN_POINT ( 'NONE',  ( -194.9999999999999432, -172.9999999999999716, 232.0000000000000284 ) ) ;
#43729=EDGE_LOOP ( 'NONE', ( #25604, #2142, #16059, #44208 ) ) ;
#43771=DIRECTION ( 'NONE',  ( 1.000000000000000000, 0.000000000000000000, 0.000000000000000000 ) ) ;
#43782=PLANE ( 'NONE',  #4526 ) ;
#43786=ORIENTED_EDGE ( 'NONE', *, *, #21454, .T. ) ;
#43789=VERTEX_POINT ( 'NONE', #33176 ) ;
#43791=CARTESIAN_POINT ( 'NONE',  ( 240.0000000000000000, -164.9999999999999716, 62.29650858650038003 ) ) ;
#43814=CARTESIAN_POINT ( 'NONE',  ( 50.00000000000000000, -50.00000000000000000, 800.0000000000000000 ) ) ;
#43817=CARTESIAN_POINT ( 'NONE',  ( 177.5000000000000000, 74.83106485270648989, -130.5992382549688955 ) ) ;
#43862=DIRECTION ( 'NONE',  ( 0.000000000000000000, -1.000000000000000000, 0.000000000000000000 ) ) ;
#43867=VECTOR ( 'NONE', #23823, 1000.000000000000000 ) ;
#43881=LINE ( 'NONE', #35202, #33271 ) ;
#43883=VERTEX_POINT ( 'NONE', #34688 ) ;
#43886=DIRECTION ( 'NONE',  ( 1.000000000000000000, -0.000000000000000000, -0.000000000000000000 ) ) ;
#43894=CARTESIAN_POINT ( 'NONE',  ( 228.9999999999999716, -169.9999999999999716, 62.29650858650038003 ) ) ;
#43895=CARTESIAN_POINT ( 'NONE',  ( 0.000000000000000000, 0.000000000000000000, 790.0000000000000000 ) ) ;
#43896=EDGE_CURVE ( 'NONE', #4645, #49554, #38294, .T. ) ;
#43902=VECTOR ( 'NONE', #25977, 1000.000000000000000 ) ;
#43922=VECTOR ( 'NONE', #18733, 1000.000000000000227 ) ;
#43966=DIRECTION ( 'NONE',  ( 1.000000000000000000, 0.000000000000000000, 0.000000000000000000 ) ) ;
#43971=ORIENTED_EDGE ( 'NONE', *, *, #43704, .T. ) ;
#43983=ORIENTED_EDGE ( 'NONE', *, *, #6186, .F. ) ;
#44018=LINE ( 'NONE', #21432, #916 ) ;
#44021=AXIS2_PLACEMENT_3D ( 'NONE', #43507, #4517, #670 ) ;
#44054=LINE ( 'NONE', #44538, #13954 ) ;
#44058=ORIENTED_EDGE ( 'NONE', *, *, #13318, .T. ) ;
#44090=VERTEX_POINT ( 'NONE', #21289 ) ;
#44106=DIRECTION ( 'NONE',  ( 0.000000000000000000, 0.9230769230769231282, 0.3846153846153844702 ) ) ;
#44172=ORIENTED_EDGE ( 'NONE', *, *, #19605, .T. ) ;
#44208=ORIENTED_EDGE ( 'NONE', *, *, #32443, .F. ) ;
#44281=PLANE ( 'NONE',  #38031 ) ;
#44286=ORIENTED_EDGE ( 'NONE', *, *, #45602, .T. ) ;
#44309=CARTESIAN_POINT ( 'NONE',  ( -177.4999999999999716, 74.83106485270648989, -130.5992382549688955 ) ) ;
#44310=FACE_OUTER_BOUND ( 'NONE', #11695, .T. ) ;
#44330=VERTEX_POINT ( 'NONE', #8689 ) ;
#44340=AXIS2_PLACEMENT_3D ( 'NONE', #39491, #234, #4329 ) ;
#44364=EDGE_CURVE ( 'NONE', #21827, #35427, #19192, .T. ) ;
#44409=ORIENTED_EDGE ( 'NONE', *, *, #3960, .F. ) ;
#44415=DIRECTION ( 'NONE',  ( 1.000000000000000000, -0.000000000000000000, -0.000000000000000000 ) ) ;
#44439=PLANE ( 'NONE',  #8641 ) ;
#44441=DIRECTION ( 'NONE',  ( 1.000000000000000000, 0.000000000000000000, 0.000000000000000000 ) ) ;
#44450=EDGE_CURVE ( 'NONE', #26268, #23532, #10382, .T. ) ;
#44460=EDGE_CURVE ( 'NONE', #23532, #10351, #5065, .T. ) ;
#44461=EDGE_CURVE ( 'NONE', #4495, #1717, #6518, .T. ) ;
#44474=CARTESIAN_POINT ( 'NONE',  ( 240.0000000000000000, -164.9999999999999716, 444.9999999999998295 ) ) ;
#44482=DIRECTION ( 'NONE',  ( 0.000000000000000000, 0.000000000000000000, -1.000000000000000000 ) ) ;
#44497=DIRECTION ( 'NONE',  ( 0.000000000000000000, 0.000000000000000000, -1.000000000000000000 ) ) ;
#44520=DIRECTION ( 'NONE',  ( 0.000000000000000000, 0.000000000000000000, -1.000000000000000000 ) ) ;
#44538=CARTESIAN_POINT ( 'NONE',  ( -194.9999999999999432, 173.0000000000000000, 252.0000000000000000 ) ) ;
#44543=CARTESIAN_POINT ( 'NONE',  ( 0.000000000000000000, -174.9999999999999147, 500.0000000000001137 ) ) ;
#44551=DIRECTION ( 'NONE',  ( -1.000000000000000000, -0.000000000000000000, -0.000000000000000000 ) ) ;
#44566=VERTEX_POINT ( 'NONE', #32549 ) ;
#44569=AXIS2_PLACEMENT_3D ( 'NONE', #23141, #38819, #46964 ) ;
#44615=VERTEX_POINT ( 'NONE', #45990 ) ;
#44621=PLANE ( 'NONE',  #14379 ) ;
#44640=EDGE_CURVE ( 'NONE', #835, #31251, #47005, .T. ) ;
#44692=CARTESIAN_POINT ( 'NONE',  ( 240.0000000000000000, -164.9999999999999716, 474.9999999999998863 ) ) ;
#44712=LINE ( 'NONE', #45202, #49148 ) ;
#44764=CARTESIAN_POINT ( 'NONE',  ( -50.00000000000000000, -50.00000000000000000, 800.0000000000000000 ) ) ;
#44785=ORIENTED_EDGE ( 'NONE', *, *, #43896, .F. ) ;
#44815=ADVANCED_FACE ( 'NONE', ( #44924 ), #10326, .T. ) ;
#44829=LINE ( 'NONE', #48907, #14803 ) ;
#44830=DIRECTION ( 'NONE',  ( 0.000000000000000000, -1.000000000000000000, 1.604368532695312981E-16 ) ) ;
#44886=VECTOR ( 'NONE', #28939, 1000.000000000000000 ) ;
#44901=ORIENTED_EDGE ( 'NONE', *, *, #15196, .T. ) ;
#44904=FACE_OUTER_BOUND ( 'NONE', #47735, .T. ) ;
#44907=CARTESIAN_POINT ( 'NONE',  ( 177.5000000000000284, 112.5000000000000000, -10.00000000000000000 ) ) ;
#44924=FACE_OUTER_BOUND ( 'NONE', #26369, .T. ) ;
#44926=EDGE_CURVE ( 'NONE', #17677, #13610, #5927, .T. ) ;
#44931=CARTESIAN_POINT ( 'NONE',  ( 177.5000000000000284, -102.5000000000000142, -10.00000000000000000 ) ) ;
#44939=PRODUCT ( 'hopper', 'hopper', '', ( #12582 ) ) ;
#44943=VERTEX_POINT ( 'NONE', #45931 ) ;
#44948=EDGE_CURVE ( 'NONE', #5026, #28864, #49765, .T. ) ;
#44949=PLANE ( 'NONE',  #46776 ) ;
#44959=VECTOR ( 'NONE', #28485, 1000.000000000000000 ) ;
#44965=VERTEX_POINT ( 'NONE', #34188 ) ;
#44977=VERTEX_POINT ( 'NONE', #46437 ) ;
#44980=DIRECTION ( 'NONE',  ( -1.000000000000000000, -0.000000000000000000, -0.000000000000000000 ) ) ;
#44988=ORIENTED_EDGE ( 'NONE', *, *, #21454, .F. ) ;
#44991=ORIENTED_EDGE ( 'NONE', *, *, #27165, .T. ) ;
#44998=ORIENTED_EDGE ( 'NONE', *, *, #18646, .T. ) ;
#45010=DIRECTION ( 'NONE',  ( -1.000000000000000000, 0.000000000000000000, -0.000000000000000000 ) ) ;
#45043=ORIENTED_EDGE ( 'NONE', *, *, #18298, .F. ) ;
#45044=FACE_BOUND ( 'NONE', #35277, .T. ) ;
#45045=CARTESIAN_POINT ( 'NONE',  ( 228.9999999999999716, -169.9999999999999716, 474.9999999999998863 ) ) ;
#45097=PLANE ( 'NONE',  #38267 ) ;
#45116=ORIENTED_EDGE ( 'NONE', *, *, #34632, .F. ) ;
#45143=EDGE_LOOP ( 'NONE', ( #6422, #32133 ) ) ;
#45166=CARTESIAN_POINT ( 'NONE',  ( 224.9999999999999432, 175.0000000000000000, 500.0000000000000000 ) ) ;
#45179=DIRECTION ( 'NONE',  ( 0.000000000000000000, -1.000000000000000000, 8.021842663476564905E-17 ) ) ;
#45180=EDGE_CURVE ( 'NONE', #18068, #44090, #5389, .T. ) ;
#45190=DIRECTION ( 'NONE',  ( 1.000000000000000000, -0.000000000000000000, -0.000000000000000000 ) ) ;
#45202=CARTESIAN_POINT ( 'NONE',  ( 194.9999999999999716, 164.9999999999999716, 500.0000000000000000 ) ) ;
#45251=PLANE ( 'NONE',  #7858 ) ;
#45277=VECTOR ( 'NONE', #3500, 1000.000000000000000 ) ;
#45309=VECTOR ( 'NONE', #15325, 1000.000000000000000 ) ;
#45330=LINE ( 'NONE', #41762, #25805 ) ;
#45368=VERTEX_POINT ( 'NONE', #12275 ) ;
#45393=PLANE ( 'NONE',  #4869 ) ;
#45421=CARTESIAN_POINT ( 'NONE',  ( 167.5000000000000000, 67.47808924524055385, -120.5992382549688955 ) ) ;
#45444=DIRECTION ( 'NONE',  ( 0.000000000000000000, -1.000000000000000000, 0.000000000000000000 ) ) ;
#45486=AXIS2_PLACEMENT_3D ( 'NONE', #31923, #7813, #35026 ) ;
#45500=DIRECTION ( 'NONE',  ( 0.000000000000000000, -0.000000000000000000, 1.000000000000000000 ) ) ;
#45531=LINE ( 'NONE', #49362, #45532 ) ;
#45532=VECTOR ( 'NONE', #14249, 1000.000000000000114 ) ;
#45535=ORIENTED_EDGE ( 'NONE', *, *, #8693, .F. ) ;
#45558=LINE ( 'NONE', #22741, #48480 ) ;
#45562=DIRECTION ( 'NONE',  ( 0.000000000000000000, 0.000000000000000000, 1.000000000000000000 ) ) ;
#45563=ADVANCED_FACE ( 'NONE', ( #48638 ), #5842, .F. ) ;
#45580=ORIENTED_EDGE ( 'NONE', *, *, #23748, .F. ) ;
#45584=EDGE_LOOP ( 'NONE', ( #41668, #15225, #24173, #26138, #39298, #12559 ) ) ;
#45597=EDGE_CURVE ( 'NONE', #16490, #12746, #18135, .T. ) ;
#45599=DIRECTION ( 'NONE',  ( 0.000000000000000000, 0.000000000000000000, 1.000000000000000000 ) ) ;
#45602=EDGE_CURVE ( 'NONE', #4602, #46359, #33810, .T. ) ;
#45632=LINE ( 'NONE', #41306, #1320 ) ;
#45657=FACE_OUTER_BOUND ( 'NONE', #17221, .T. ) ;
#45669=CARTESIAN_POINT ( 'NONE',  ( 167.5000000000000000, -112.5000000000000000, -10.00000000000000000 ) ) ;
#45675=ORIENTED_EDGE ( 'NONE', *, *, #44450, .T. ) ;
#45694=LINE ( 'NONE', #25477, #10517 ) ;
#45696=EDGE_CURVE ( 'NONE', #42074, #48180, #8384, .T. ) ;
#45707=EDGE_CURVE ( 'NONE', #22662, #9652, #47072, .T. ) ;
#45719=AXIS2_PLACEMENT_3D ( 'NONE', #33940, #48785, #17277 ) ;
#45725=ORIENTED_EDGE ( 'NONE', *, *, #25355, .F. ) ;
#45732=ORIENTED_EDGE ( 'NONE', *, *, #26524, .T. ) ;
#45741=ORIENTED_EDGE ( 'NONE', *, *, #10217, .F. ) ;
#45761=VECTOR ( 'NONE', #11257, 1000.000000000000000 ) ;
#45767=LINE ( 'NONE', #14753, #13366 ) ;
#45769=DIRECTION ( 'NONE',  ( 0.000000000000000000, 1.000000000000000000, -2.406552799042969348E-16 ) ) ;
#45772=DIRECTION ( 'NONE',  ( 0.000000000000000000, 0.000000000000000000, 1.000000000000000000 ) ) ;
#45788=VECTOR ( 'NONE', #42380, 1000.000000000000000 ) ;
#45795=ORIENTED_EDGE ( 'NONE', *, *, #28462, .F. ) ;
#45802=CARTESIAN_POINT ( 'NONE',  ( 0.000000000000000000, -72.49999999999998579, 0.000000000000000000 ) ) ;
#45803=LINE ( 'NONE', #26350, #30918 ) ;
#45831=VECTOR ( 'NONE', #5673, 1000.000000000000000 ) ;
#45834=CARTESIAN_POINT ( 'NONE',  ( 214.9999999999999432, -172.9999999999999716, 232.0000000000000284 ) ) ;
#45838=DIRECTION ( 'NONE',  ( 0.000000000000000000, 1.000000000000000000, -1.604368532695312981E-16 ) ) ;
#45873=DIRECTION ( 'NONE',  ( 0.000000000000000000, 0.000000000000000000, -1.000000000000000000 ) ) ;
#45874=CARTESIAN_POINT ( 'NONE',  ( 177.5000000000000000, 74.83106485270648989, -130.5992382549688955 ) ) ;
#45902=ORIENTED_EDGE ( 'NONE', *, *, #33734, .T. ) ;
#45903=CARTESIAN_POINT ( 'NONE',  ( 224.9999999999999716, -175.0000000000000000, 499.9999999999998863 ) ) ;
#45908=LINE ( 'NONE', #30551, #36566 ) ;
#45910=AXIS2_PLACEMENT_3D ( 'NONE', #50258, #15170, #22351 ) ;
#45931=CARTESIAN_POINT ( 'NONE',  ( -21.24469349090191983, 33.89193117067290473, 910.0000000000000000 ) ) ;
#45932=EDGE_LOOP ( 'NONE', ( #11179, #28903, #24446, #32461 ) ) ;
#45939=EDGE_CURVE ( 'NONE', #5061, #19653, #2925, .T. ) ;
#45951=DIRECTION ( 'NONE',  ( -0.000000000000000000, -0.000000000000000000, 1.000000000000000000 ) ) ;
#45963=VERTEX_POINT ( 'NONE', #2192 ) ;
#45972=ORIENTED_EDGE ( 'NONE', *, *, #10025, .T. ) ;
#45975=DIRECTION ( 'NONE',  ( -0.4055129968046615185, -0.4055129968046615185, -0.8192181753629523833 ) ) ;
#45976=CARTESIAN_POINT ( 'NONE',  ( 102.1135063278031652, 164.9999999999999716, 690.8162120245517599 ) ) ;
#45986=ORIENTED_EDGE ( 'NONE', *, *, #23372, .T. ) ;
#45990=CARTESIAN_POINT ( 'NONE',  ( -581.3085477938157055, 47.50000000000000000, -68.52876838486925237 ) ) ;
#46052=CYLINDRICAL_SURFACE ( 'NONE', #10450, 3.500000000000003109 ) ;
#46103=VERTEX_POINT ( 'NONE', #4888 ) ;
#46105=VECTOR ( 'NONE', #4276, 1000.000000000000227 ) ;
#46184=DIRECTION ( 'NONE',  ( -1.000000000000000000, 0.000000000000000000, 0.000000000000000000 ) ) ;
#46185=CARTESIAN_POINT ( 'NONE',  ( 325.0507910275983932, 325.0507910275983932, 321.8002831173224649 ) ) ;
#46192=DIRECTION ( 'NONE',  ( -0.000000000000000000, 1.000000000000000000, -2.406552799042969348E-16 ) ) ;
#46196=CARTESIAN_POINT ( 'NONE',  ( 376.8544389702901753, 0.000000000000000000, 219.8317560660024697 ) ) ;
#46257=CARTESIAN_POINT ( 'NONE',  ( -194.9999999999999432, -172.9999999999999716, 232.0000000000000284 ) ) ;
#46260=VECTOR ( 'NONE', #36142, 1000.000000000000000 ) ;
#46261=CARTESIAN_POINT ( 'NONE',  ( -225.0000000000000568, 164.9999999999999716, 352.0000000000000000 ) ) ;
#46266=EDGE_LOOP ( 'NONE', ( #39363, #21580, #49486, #46607, #41821 ) ) ;
#46268=DIRECTION ( 'NONE',  ( 0.000000000000000000, -2.406552799042969348E-16, -1.000000000000000000 ) ) ;
#46288=ORIENTED_EDGE ( 'NONE', *, *, #28678, .F. ) ;
#46292=AXIS2_PLACEMENT_3D ( 'NONE', #11146, #11388, #47007 ) ;
#46318=VECTOR ( 'NONE', #18556, 1000.000000000000000 ) ;
#46349=CARTESIAN_POINT ( 'NONE',  ( -214.9999999999999432, -173.0000000000000000, 352.0000000000000568 ) ) ;
#46354=ORIENTED_EDGE ( 'NONE', *, *, #18008, .T. ) ;
#46355=CARTESIAN_POINT ( 'NONE',  ( 50.00000000000000000, -50.00000000000000000, 800.0000000000000000 ) ) ;
#46359=VERTEX_POINT ( 'NONE', #19468 ) ;
#46389=CARTESIAN_POINT ( 'NONE',  ( -50.00000000000000000, 50.00000000000000000, 800.0000000000000000 ) ) ;
#46407=EDGE_LOOP ( 'NONE', ( #40975, #30957, #10811, #32854, #5057, #19999 ) ) ;
#46426=ORIENTED_EDGE ( 'NONE', *, *, #5254, .F. ) ;
#46437=CARTESIAN_POINT ( 'NONE',  ( -215.0000000000000568, -173.0000000000000000, 372.0000000000000000 ) ) ;
#46514=LINE ( 'NONE', #3957, #33897 ) ;
#46517=ORIENTED_EDGE ( 'NONE', *, *, #18007, .T. ) ;
#46548=ORIENTED_EDGE ( 'NONE', *, *, #24041, .T. ) ;
#46579=ORIENTED_EDGE ( 'NONE', *, *, #21532, .F. ) ;
#46607=ORIENTED_EDGE ( 'NONE', *, *, #41238, .F. ) ;
#46620=CARTESIAN_POINT ( 'NONE',  ( 214.9999999999999432, -173.0000000000000000, 372.0000000000000000 ) ) ;
#46664=CARTESIAN_POINT ( 'NONE',  ( 177.5000000000000284, 102.5000000000000142, -10.00000000000000000 ) ) ;
#46697=DIRECTION ( 'NONE',  ( 0.000000000000000000, -1.000000000000000000, 0.000000000000000000 ) ) ;
#46725=DIRECTION ( 'NONE',  ( 0.000000000000000000, 0.000000000000000000, 1.000000000000000000 ) ) ;
#46740=ORIENTED_EDGE ( 'NONE', *, *, #4887, .T. ) ;
#46757=DIRECTION ( 'NONE',  ( 0.000000000000000000, 0.000000000000000000, 1.000000000000000000 ) ) ;
#46761=CARTESIAN_POINT ( 'NONE',  ( 44.25629667545848633, 43.33333333333339255, 790.0000000000000000 ) ) ;
#46776=AXIS2_PLACEMENT_3D ( 'NONE', #33455, #13919, #29587 ) ;
#46793=CARTESIAN_POINT ( 'NONE',  ( -33.89193117067290473, -21.24469349090191983, 910.0000000000000000 ) ) ;
#46797=EDGE_CURVE ( 'NONE', #50400, #21827, #9858, .T. ) ;
#46813=CARTESIAN_POINT ( 'NONE',  ( 0.000000000000000000, -317.3964497041420145, 132.2485207100591253 ) ) ;
#46828=CARTESIAN_POINT ( 'NONE',  ( 232.4999999999999716, -169.9999999999999716, 474.9999999999998863 ) ) ;
#46842=ORIENTED_EDGE ( 'NONE', *, *, #1700, .F. ) ;
#46857=EDGE_CURVE ( 'NONE', #45963, #38992, #25018, .T. ) ;
#46874=PLANE ( 'NONE',  #44340 ) ;
#46884=CARTESIAN_POINT ( 'NONE',  ( -167.4999999999999716, 102.9547873477646647, -7.018571579996165433 ) ) ;
#46897=EDGE_LOOP ( 'NONE', ( #49736, #1708, #24374 ) ) ;
#46929=ORIENTED_EDGE ( 'NONE', *, *, #1451, .F. ) ;
#46964=DIRECTION ( 'NONE',  ( 1.000000000000000000, 0.000000000000000000, 0.000000000000000000 ) ) ;
#46993=EDGE_CURVE ( 'NONE', #16851, #50400, #33132, .T. ) ;
#46995=EDGE_CURVE ( 'NONE', #47971, #35326, #12353, .T. ) ;
#46996=CARTESIAN_POINT ( 'NONE',  ( -582.5000000000000000, 57.49999999999996447, -58.60000000000003695 ) ) ;
#47005=LINE ( 'NONE', #106, #47678 ) ;
#47007=DIRECTION ( 'NONE',  ( 0.000000000000000000, -1.000000000000000000, 1.604368532695312981E-16 ) ) ;
#47008=ORIENTED_EDGE ( 'NONE', *, *, #9273, .T. ) ;
#47016=DIRECTION ( 'NONE',  ( -1.000000000000000000, 0.000000000000000000, 0.000000000000000000 ) ) ;
#47038=VECTOR ( 'NONE', #44441, 1000.000000000000000 ) ;
#47047=ORIENTED_EDGE ( 'NONE', *, *, #43704, .F. ) ;
#47072=LINE ( 'NONE', #19912, #45309 ) ;
#47077=CARTESIAN_POINT ( 'NONE',  ( 40.00000000000000000, 4.898587196589413026E-15, 790.0000000000000000 ) ) ;
#47084=VECTOR ( 'NONE', #48518, 1000.000000000000000 ) ;
#47086=AXIS2_PLACEMENT_3D ( 'NONE', #707, #16357, #32023 ) ;
#47134=LINE ( 'NONE', #8188, #35929 ) ;
#47184=CARTESIAN_POINT ( 'NONE',  ( -167.4999999999999716, 74.83106485270648989, -120.5992382549688955 ) ) ;
#47201=VECTOR ( 'NONE', #15666, 1000.000000000000000 ) ;
#47245=CARTESIAN_POINT ( 'NONE',  ( 432.7825420346616170, 47.50000000000000000, -120.5992382549688955 ) ) ;
#47300=LINE ( 'NONE', #50444, #14669 ) ;
#47313=CARTESIAN_POINT ( 'NONE',  ( 224.9999999999999432, -175.0000000000000000, 444.9999999999998295 ) ) ;
#47314=ADVANCED_FACE ( 'NONE', ( #17959 ), #23081, .T. ) ;
#47319=ORIENTED_EDGE ( 'NONE', *, *, #34632, .T. ) ;
#47322=LINE ( 'NONE', #19655, #36291 ) ;
#47325=CYLINDRICAL_SURFACE ( 'NONE', #44021, 40.00000000000000000 ) ;
#47350=CARTESIAN_POINT ( 'NONE',  ( -239.0000000000000853, 0.000000000000000000, 0.000000000000000000 ) ) ;
#47387=LINE ( 'NONE', #24105, #5688 ) ;
#47445=AXIS2_PLACEMENT_3D ( 'NONE', #41476, #29933, #22977 ) ;
#47459=CARTESIAN_POINT ( 'NONE',  ( -385.4922279792746167, 0.000000000000000000, 224.8704663212436117 ) ) ;
#47467=EDGE_CURVE ( 'NONE', #29654, #34586, #12295, .T. ) ;
#47486=DIRECTION ( 'NONE',  ( -1.000000000000000000, 0.000000000000000000, -0.000000000000000000 ) ) ;
#47487=VECTOR ( 'NONE', #6642, 1000.000000000000000 ) ;
#47503=EDGE_CURVE ( 'NONE', #18068, #20648, #4839, .T. ) ;
#47519=AXIS2_PLACEMENT_3D ( 'NONE', #34265, #26817, #42449 ) ;
#47530=CARTESIAN_POINT ( 'NONE',  ( -177.4999999999999716, 57.49999999999996447, -9.999999999999973355 ) ) ;
#47557=AXIS2_PLACEMENT_3D ( 'NONE', #38120, #14751, #45010 ) ;
#47565=VERTEX_POINT ( 'NONE', #13045 ) ;
#47590=DIRECTION ( 'NONE',  ( 0.000000000000000000, -1.604368532695312981E-16, -1.000000000000000000 ) ) ;
#47601=ORIENTED_EDGE ( 'NONE', *, *, #6428, .T. ) ;
#47622=EDGE_LOOP ( 'NONE', ( #5156, #3531, #26166, #49532 ) ) ;
#47632=DIRECTION ( 'NONE',  ( -0.000000000000000000, 1.000000000000000000, -1.604368532695312981E-16 ) ) ;
#47636=LINE ( 'NONE', #28685, #16025 ) ;
#47645=CARTESIAN_POINT ( 'NONE',  ( 214.9999999999999432, 164.9999999999999716, 500.0000000000000000 ) ) ;
#47655=DIRECTION ( 'NONE',  ( 0.000000000000000000, -1.000000000000000000, 8.021842663476564905E-17 ) ) ;
#47661=ORIENTED_EDGE ( 'NONE', *, *, #11528, .F. ) ;
#47670=EDGE_LOOP ( 'NONE', ( #3695, #23222, #13458, #20426 ) ) ;
#47673=CARTESIAN_POINT ( 'NONE',  ( 240.0000000000000000, -175.0000000000000000, 474.9999999999998863 ) ) ;
#47678=VECTOR ( 'NONE', #38607, 1000.000000000000000 ) ;
#47722=EDGE_CURVE ( 'NONE', #3623, #14442, #3255, .T. ) ;
#47733=DIRECTION ( 'NONE',  ( 0.000000000000000000, 0.000000000000000000, -1.000000000000000000 ) ) ;
#47735=EDGE_LOOP ( 'NONE', ( #31023, #4206, #26396, #5602, #7819 ) ) ;
#47739=CARTESIAN_POINT ( 'NONE',  ( -582.5000000000000000, 57.49999999999996447, -58.60000000000003695 ) ) ;
#47777=ADVANCED_FACE ( 'NONE', ( #38690 ), #31249, .F. ) ;
#47782=ADVANCED_FACE ( 'NONE', ( #15836, #43019 ), #19429, .T. ) ;
#47808=ORIENTED_EDGE ( 'NONE', *, *, #20260, .T. ) ;
#47814=ORIENTED_EDGE ( 'NONE', *, *, #29081, .T. ) ;
#47847=VECTOR ( 'NONE', #26916, 1000.000000000000227 ) ;
#47873=FACE_OUTER_BOUND ( 'NONE', #9987, .T. ) ;
#47876=ORIENTED_EDGE ( 'NONE', *, *, #13368, .T. ) ;
#47877=ORIENTED_EDGE ( 'NONE', *, *, #40862, .F. ) ;
#47907=EDGE_LOOP ( 'NONE', ( #45043, #18931, #18045, #9660 ) ) ;
#47923=CARTESIAN_POINT ( 'NONE',  ( 240.0000000000000000, -164.9999999999999716, 32.29650858650035161 ) ) ;
#47971=VERTEX_POINT ( 'NONE', #49103 ) ;
#48005=VERTEX_POINT ( 'NONE', #7781 ) ;
#48033=ORIENTED_EDGE ( 'NONE', *, *, #36701, .T. ) ;
#48070=CARTESIAN_POINT ( 'NONE',  ( 177.5000000000000000, -77.43746236555679729, -130.5992382549688671 ) ) ;
#48081=DIRECTION ( 'NONE',  ( 0.000000000000000000, 1.000000000000000000, -0.000000000000000000 ) ) ;
#48128=DIRECTION ( 'NONE',  ( 0.000000000000000000, 1.000000000000000000, 0.000000000000000000 ) ) ;
#48138=FACE_OUTER_BOUND ( 'NONE', #43729, .T. ) ;
#48140=EDGE_CURVE ( 'NONE', #8986, #10351, #8534, .T. ) ;
#48141=DIRECTION ( 'NONE',  ( -0.9928768384869219865, 0.000000000000000000, -0.1191452206184307749 ) ) ;
#48177=VERTEX_POINT ( 'NONE', #15975 ) ;
#48178=CARTESIAN_POINT ( 'NONE',  ( -214.9999999999999432, -173.0000000000000000, 352.0000000000000568 ) ) ;
#48180=VERTEX_POINT ( 'NONE', #32382 ) ;
#48214=DIRECTION ( 'NONE',  ( -0.8637789008984334549, 0.000000000000000000, 0.5038710255240862468 ) ) ;
#48226=ORIENTED_EDGE ( 'NONE', *, *, #5443, .F. ) ;
#48246=AXIS2_PLACEMENT_3D ( 'NONE', #27920, #32281, #43555 ) ;
#48250=LINE ( 'NONE', #45166, #43131 ) ;
#48258=CARTESIAN_POINT ( 'NONE',  ( 385.4922279792745030, 0.000000000000000000, 224.8704663212433275 ) ) ;
#48260=ORIENTED_EDGE ( 'NONE', *, *, #1451, .T. ) ;
#48262=ORIENTED_EDGE ( 'NONE', *, *, #32443, .T. ) ;
#48298=EDGE_LOOP ( 'NONE', ( #24937, #8150, #12708, #26776, #7094 ) ) ;
#48312=VECTOR ( 'NONE', #31372, 1000.000000000000000 ) ;
#48320=ORIENTED_EDGE ( 'NONE', *, *, #47467, .F. ) ;
#48345=VECTOR ( 'NONE', #40399, 1000.000000000000000 ) ;
#48352=DIRECTION ( 'NONE',  ( -1.000000000000000000, 0.000000000000000000, 0.000000000000000000 ) ) ;
#48371=CARTESIAN_POINT ( 'NONE',  ( -177.4999999999999716, 112.5000000000000000, -10.00000000000000000 ) ) ;
#48398=CARTESIAN_POINT ( 'NONE',  ( -567.5000000000000000, 57.49999999999996447, -183.5999999999997954 ) ) ;
#48417=VERTEX_POINT ( 'NONE', #42079 ) ;
#48422=EDGE_CURVE ( 'NONE', #22675, #13610, #22331, .T. ) ;
#48429=FACE_OUTER_BOUND ( 'NONE', #36369, .T. ) ;
#48447=CARTESIAN_POINT ( 'NONE',  ( 50.00000000000000000, -50.00000000000000000, 800.0000000000000000 ) ) ;
#48457=VECTOR ( 'NONE', #46697, 1000.000000000000000 ) ;
#48480=VECTOR ( 'NONE', #14792, 1000.000000000000000 ) ;
#48496=CARTESIAN_POINT ( 'NONE',  ( -33.89193117067293315, 33.89193117067293315, 910.0000000000000000 ) ) ;
#48508=LINE ( 'NONE', #29311, #25902 ) ;
#48518=DIRECTION ( 'NONE',  ( 0.000000000000000000, -1.000000000000000000, 0.000000000000000000 ) ) ;
#48523=FACE_OUTER_BOUND ( 'NONE', #5697, .T. ) ;
#48541=VECTOR ( 'NONE', #422, 1000.000000000000000 ) ;
#48565=FACE_OUTER_BOUND ( 'NONE', #27804, .T. ) ;
#48598=CARTESIAN_POINT ( 'NONE',  ( 167.5000000000000000, -102.5000000000000142, -10.00000000000000000 ) ) ;
#48606=ORIENTED_EDGE ( 'NONE', *, *, #5477, .F. ) ;
#48634=DIRECTION ( 'NONE',  ( -1.000000000000000000, 0.000000000000000000, 0.000000000000000000 ) ) ;
#48638=FACE_OUTER_BOUND ( 'NONE', #39873, .T. ) ;
#48645=LINE ( 'NONE', #41750, #1602 ) ;
#48660=VERTEX_POINT ( 'NONE', #13803 ) ;
#48666=ORIENTED_EDGE ( 'NONE', *, *, #8874, .T. ) ;
#48670=DIRECTION ( 'NONE',  ( 0.8962124318248270161, -0.000000000000000000, 0.4436251537532894806 ) ) ;
#48693=VECTOR ( 'NONE', #30170, 1000.000000000000000 ) ;
#48722=CARTESIAN_POINT ( 'NONE',  ( -225.0000000000000568, 164.9999999999999716, 500.0000000000000000 ) ) ;
#48784=ADVANCED_FACE ( 'NONE', ( #14572 ), #26885, .F. ) ;
#48785=DIRECTION ( 'NONE',  ( 0.000000000000000000, 1.000000000000000000, 0.000000000000000000 ) ) ;
#48806=CARTESIAN_POINT ( 'NONE',  ( 0.000000000000000000, 50.00000000000000000, 900.0000000000000000 ) ) ;
#48836=CARTESIAN_POINT ( 'NONE',  ( -44.25629667545849344, 43.33333333333339255, 790.0000000000000000 ) ) ;
#48864=DIRECTION ( 'NONE',  ( 0.000000000000000000, 1.000000000000000000, -0.000000000000000000 ) ) ;
#48873=CARTESIAN_POINT ( 'NONE',  ( 37.90972275097263378, -14.83505920947803780, 901.8832493327278144 ) ) ;
#48886=LINE ( 'NONE', #24840, #41296 ) ;
#48907=CARTESIAN_POINT ( 'NONE',  ( -214.9999999999999432, 173.0000000000000000, 252.0000000000000000 ) ) ;
#48917=DIRECTION ( 'NONE',  ( 1.000000000000000000, -0.000000000000000000, 0.000000000000000000 ) ) ;
#48944=EDGE_LOOP ( 'NONE', ( #21608, #5805, #1346, #27020 ) ) ;
#48949=ORIENTED_EDGE ( 'NONE', *, *, #41354, .F. ) ;
#48960=AXIS2_PLACEMENT_3D ( 'NONE', #1995, #34069, #2992 ) ;
#48961=EDGE_LOOP ( 'NONE', ( #42018, #41854, #6315, #46842 ) ) ;
#48991=ADVANCED_FACE ( 'NONE', ( #8903 ), #44281, .F. ) ;
#49050=AXIS2_PLACEMENT_3D ( 'NONE', #27002, #35484, #27267 ) ;
#49065=PLANE ( 'NONE',  #11975 ) ;
#49070=CARTESIAN_POINT ( 'NONE',  ( 194.9999999999999432, -172.9999999999999716, 232.0000000000000284 ) ) ;
#49096=EDGE_CURVE ( 'NONE', #21827, #7894, #18107, .T. ) ;
#49103=CARTESIAN_POINT ( 'NONE',  ( -215.0000000000000568, -175.0000000000000000, 474.0000000000000000 ) ) ;
#49107=AXIS2_PLACEMENT_3D ( 'NONE', #528, #7712, #20004 ) ;
#49132=ORIENTED_EDGE ( 'NONE', *, *, #21153, .F. ) ;
#49148=VECTOR ( 'NONE', #6254, 1000.000000000000000 ) ;
#49237=DIRECTION ( 'NONE',  ( -0.000000000000000000, -0.000000000000000000, 1.000000000000000000 ) ) ;
#49267=LINE ( 'NONE', #25722, #7824 ) ;
#49269=EDGE_CURVE ( 'NONE', #1551, #6362, #34803, .T. ) ;
#49286=VERTEX_POINT ( 'NONE', #44474 ) ;
#49296=CARTESIAN_POINT ( 'NONE',  ( 194.9999999999999432, 173.0000000000000000, 372.0000000000000000 ) ) ;
#49303=EDGE_LOOP ( 'NONE', ( #41595, #49132, #48320, #38977 ) ) ;
#49308=VERTEX_POINT ( 'NONE', #29107 ) ;
#49323=CARTESIAN_POINT ( 'NONE',  ( 50.00000000000000000, -50.00000000000000000, 900.0000000000000000 ) ) ;
#49348=CARTESIAN_POINT ( 'NONE',  ( -194.9999999999999432, -172.9999999999999716, 232.0000000000000284 ) ) ;
#49353=ORIENTED_EDGE ( 'NONE', *, *, #12405, .T. ) ;
#49362=CARTESIAN_POINT ( 'NONE',  ( 0.5000000000000000000, -0.5000000000000000000, 1000.000000000000000 ) ) ;
#49388=ORIENTED_EDGE ( 'NONE', *, *, #3828, .T. ) ;
#49409=CARTESIAN_POINT ( 'NONE',  ( 0.000000000000000000, 0.000000000000000000, 800.0000000000000000 ) ) ;
#49421=CARTESIAN_POINT ( 'NONE',  ( 224.9999999999999716, -164.9999999999999716, 62.29650858650038003 ) ) ;
#49424=CARTESIAN_POINT ( 'NONE',  ( -225.0000000000000284, -174.9999999999999716, 500.0000000000001137 ) ) ;
#49432=CARTESIAN_POINT ( 'NONE',  ( 0.5000000000000000000, 0.5000000000000000000, 1000.000000000000000 ) ) ;
#49440=DIRECTION ( 'NONE',  ( 0.000000000000000000, 1.000000000000000000, 0.000000000000000000 ) ) ;
#49442=LINE ( 'NONE', #6636, #40716 ) ;
#49466=VECTOR ( 'NONE', #33780, 1000.000000000000000 ) ;
#49469=ORIENTED_EDGE ( 'NONE', *, *, #13464, .F. ) ;
#49475=( NAMED_UNIT ( * ) SI_UNIT ( $, .STERADIAN. ) SOLID_ANGLE_UNIT ( ) );
#49481=DIRECTION ( 'NONE',  ( 0.000000000000000000, 0.000000000000000000, 1.000000000000000000 ) ) ;
#49486=ORIENTED_EDGE ( 'NONE', *, *, #40330, .F. ) ;
#49514=DIRECTION ( 'NONE',  ( 0.4436251537532894806, 0.000000000000000000, 0.8962124318248270161 ) ) ;
#49528=DIRECTION ( 'NONE',  ( 0.000000000000000000, -0.000000000000000000, -1.000000000000000000 ) ) ;
#49532=ORIENTED_EDGE ( 'NONE', *, *, #3700, .T. ) ;
#49541=DIRECTION ( 'NONE',  ( -0.000000000000000000, -1.000000000000000000, -0.000000000000000000 ) ) ;
#49554=VERTEX_POINT ( 'NONE', #43420 ) ;
#49577=CARTESIAN_POINT ( 'NONE',  ( 214.9999999999999432, 173.0000000000000000, 252.0000000000000000 ) ) ;
#49580=LINE ( 'NONE', #25783, #9557 ) ;
#49589=DIRECTION ( 'NONE',  ( 0.000000000000000000, 0.000000000000000000, -1.000000000000000000 ) ) ;
#49597=VECTOR ( 'NONE', #35802, 999.9999999999998863 ) ;
#49618=VERTEX_POINT ( 'NONE', #31655 ) ;
#49651=DIRECTION ( 'NONE',  ( 1.000000000000000000, 0.000000000000000000, 0.000000000000000000 ) ) ;
#49656=EDGE_CURVE ( 'NONE', #9673, #2521, #40099, .T. ) ;
#49662=LINE ( 'NONE', #33565, #41078 ) ;
#49665=LINE ( 'NONE', #15069, #45277 ) ;
#49672=ORIENTED_EDGE ( 'NONE', *, *, #718, .F. ) ;
#49684=DIRECTION ( 'NONE',  ( 0.000000000000000000, -1.604368532695312981E-16, -1.000000000000000000 ) ) ;
#49725=CARTESIAN_POINT ( 'NONE',  ( 0.000000000000000000, 0.000000000000000000, 900.0000000000000000 ) ) ;
#49736=ORIENTED_EDGE ( 'NONE', *, *, #13313, .F. ) ;
#49750=ORIENTED_EDGE ( 'NONE', *, *, #17486, .T. ) ;
#49765=LINE ( 'NONE', #30840, #41159 ) ;
#49840=EDGE_CURVE ( 'NONE', #1605, #1551, #2775, .T. ) ;
#49842=CARTESIAN_POINT ( 'NONE',  ( 177.5000000000000284, -112.5000000000000000, 0.000000000000000000 ) ) ;
#49856=EDGE_LOOP ( 'NONE', ( #2031, #23790, #32731, #11378, #32610, #24443 ) ) ;
#49861=AXIS2_PLACEMENT_3D ( 'NONE', #42006, #38430, #26613 ) ;
#49874=DIRECTION ( 'NONE',  ( -1.000000000000000000, 0.000000000000000000, 0.000000000000000000 ) ) ;
#49875=CARTESIAN_POINT ( 'NONE',  ( 50.00000000000000000, 50.00000000000000000, 800.0000000000000000 ) ) ;
#49879=PLANE ( 'NONE',  #38921 ) ;
#49884=ORIENTED_EDGE ( 'NONE', *, *, #36761, .T. ) ;
#49914=EDGE_CURVE ( 'NONE', #39676, #16604, #18424, .T. ) ;
#49917=ORIENTED_EDGE ( 'NONE', *, *, #34728, .T. ) ;
#49938=ORIENTED_EDGE ( 'NONE', *, *, #42565, .F. ) ;
#49958=VECTOR ( 'NONE', #50462, 1000.000000000000114 ) ;
#49973=ORIENTED_EDGE ( 'NONE', *, *, #6548, .T. ) ;
#49988=ORIENTED_EDGE ( 'NONE', *, *, #24112, .T. ) ;
#49990=DIRECTION ( 'NONE',  ( -0.000000000000000000, -0.000000000000000000, -1.000000000000000000 ) ) ;
#50032=ADVANCED_FACE ( 'NONE', ( #19944 ), #39724, .T. ) ;
#50035=ORIENTED_EDGE ( 'NONE', *, *, #47467, .T. ) ;
#50059=CARTESIAN_POINT ( 'NONE',  ( -225.0000000000000568, -175.0000000000000000, 500.0000000000000000 ) ) ;
#50072=ORIENTED_EDGE ( 'NONE', *, *, #6928, .F. ) ;
#50102=EDGE_LOOP ( 'NONE', ( #33475, #50613, #38914, #22835 ) ) ;
#50112=VERTEX_POINT ( 'NONE', #33029 ) ;
#50156=DIRECTION ( 'NONE',  ( -0.000000000000000000, -0.000000000000000000, 1.000000000000000000 ) ) ;
#50208=AXIS2_PLACEMENT_3D ( 'NONE', #48258, #21101, #612 ) ;
#50216=( NAMED_UNIT ( * ) PLANE_ANGLE_UNIT ( ) SI_UNIT ( $, .RADIAN. ) );
#50225=EDGE_CURVE ( 'NONE', #639, #2566, #42227, .T. ) ;
#50258=CARTESIAN_POINT ( 'NONE',  ( 232.4999999999999716, -169.9999999999999716, 4.999999999999616307 ) ) ;
#50265=PLANE ( 'NONE',  #40894 ) ;
#50272=VECTOR ( 'NONE', #25149, 1000.000000000000000 ) ;
#50298=ORIENTED_EDGE ( 'NONE', *, *, #18938, .T. ) ;
#50323=CIRCLE ( 'NONE', #17631, 40.00000000000000000 ) ;
#50339=ORIENTED_EDGE ( 'NONE', *, *, #26448, .T. ) ;
#50347=ORIENTED_EDGE ( 'NONE', *, *, #16741, .F. ) ;
#50397=DIRECTION ( 'NONE',  ( 1.341289691698241816E-15, -1.000000000000000000, 1.822804496942679766E-16 ) ) ;
#50400=VERTEX_POINT ( 'NONE', #13178 ) ;
#50424=VECTOR ( 'NONE', #22156, 1000.000000000000000 ) ;
#50428=ORIENTED_EDGE ( 'NONE', *, *, #41760, .F. ) ;
#50444=CARTESIAN_POINT ( 'NONE',  ( -194.9999999999999432, -173.0000000000000000, 352.0000000000000568 ) ) ;
#50450=VECTOR ( 'NONE', #5942, 1000.000000000000000 ) ;
#50462=DIRECTION ( 'NONE',  ( 0.1191452206184309831, 0.000000000000000000, -0.9928768384869219865 ) ) ;
#50495=VECTOR ( 'NONE', #37696, 1000.000000000000000 ) ;
#50514=ORIENTED_EDGE ( 'NONE', *, *, #46993, .F. ) ;
#50535=CARTESIAN_POINT ( 'NONE',  ( -33.89193117067290473, 0.000000000000000000, 910.0000000000000000 ) ) ;
#50551=EDGE_CURVE ( 'NONE', #50112, #29800, #26401, .T. ) ;
#50561=DIRECTION ( 'NONE',  ( 0.000000000000000000, -0.3846153846153844702, 0.9230769230769231282 ) ) ;
#50582=EDGE_LOOP ( 'NONE', ( #3424, #19382, #21924, #41023 ) ) ;
#50597=( LENGTH_UNIT ( ) NAMED_UNIT ( * ) SI_UNIT ( .MILLI., .METRE. ) );
#50598=DIRECTION ( 'NONE',  ( 0.000000000000000000, 1.000000000000000000, -8.021842663476564905E-17 ) ) ;
#50608=PLANE ( 'NONE',  #28339 ) ;
#50613=ORIENTED_EDGE ( 'NONE', *, *, #17459, .F. ) ;
#50625=ORIENTED_EDGE ( 'NONE', *, *, #45180, .F. ) ;
#50626=CARTESIAN_POINT ( 'NONE',  ( 167.5000000000000000, 102.5000000000000142, -8.474599139414886295 ) ) ;
#50630=ORIENTED_EDGE ( 'NONE', *, *, #29279, .T. ) ;
#50639=CARTESIAN_POINT ( 'NONE',  ( -40.00000000000000000, -7.564790863224938100, 897.6604670114604687 ) ) ;
#50655=VECTOR ( 'NONE', #37104, 1000.000000000000000 ) ;
#50658=LINE ( 'NONE', #11707, #39996 ) ;
#50680=FACE_OUTER_BOUND ( 'NONE', #9726, .T. ) ;
#50681=DIRECTION ( 'NONE',  ( 0.000000000000000000, 0.000000000000000000, -1.000000000000000000 ) ) ;
#50686=ORIENTED_EDGE ( 'NONE', *, *, #24357, .T. ) ;
#50708=EDGE_LOOP ( 'NONE', ( #46579, #24388, #19744, #22246 ) ) ;
#50716=CARTESIAN_POINT ( 'NONE',  ( 0.000000000000000000, 47.50000000000000000, 0.000000000000000000 ) ) ;
#50748=COLOUR_RGB('Light Blue',0.38,0.62,0.78);
#50749=FILL_AREA_STYLE_COLOUR('',#50748);
#50750=FILL_AREA_STYLE('',(#50749));
#50751=SURFACE_STYLE_FILL_AREA(#50750);
#50752=SURFACE_SIDE_STYLE('',(#50751));
#50753=SURFACE_STYLE_USAGE(.BOTH.,#50752);
#50754=PRESENTATION_STYLE_ASSIGNMENT((#50753));
ENDSEC;
END-ISO-10303-21;
